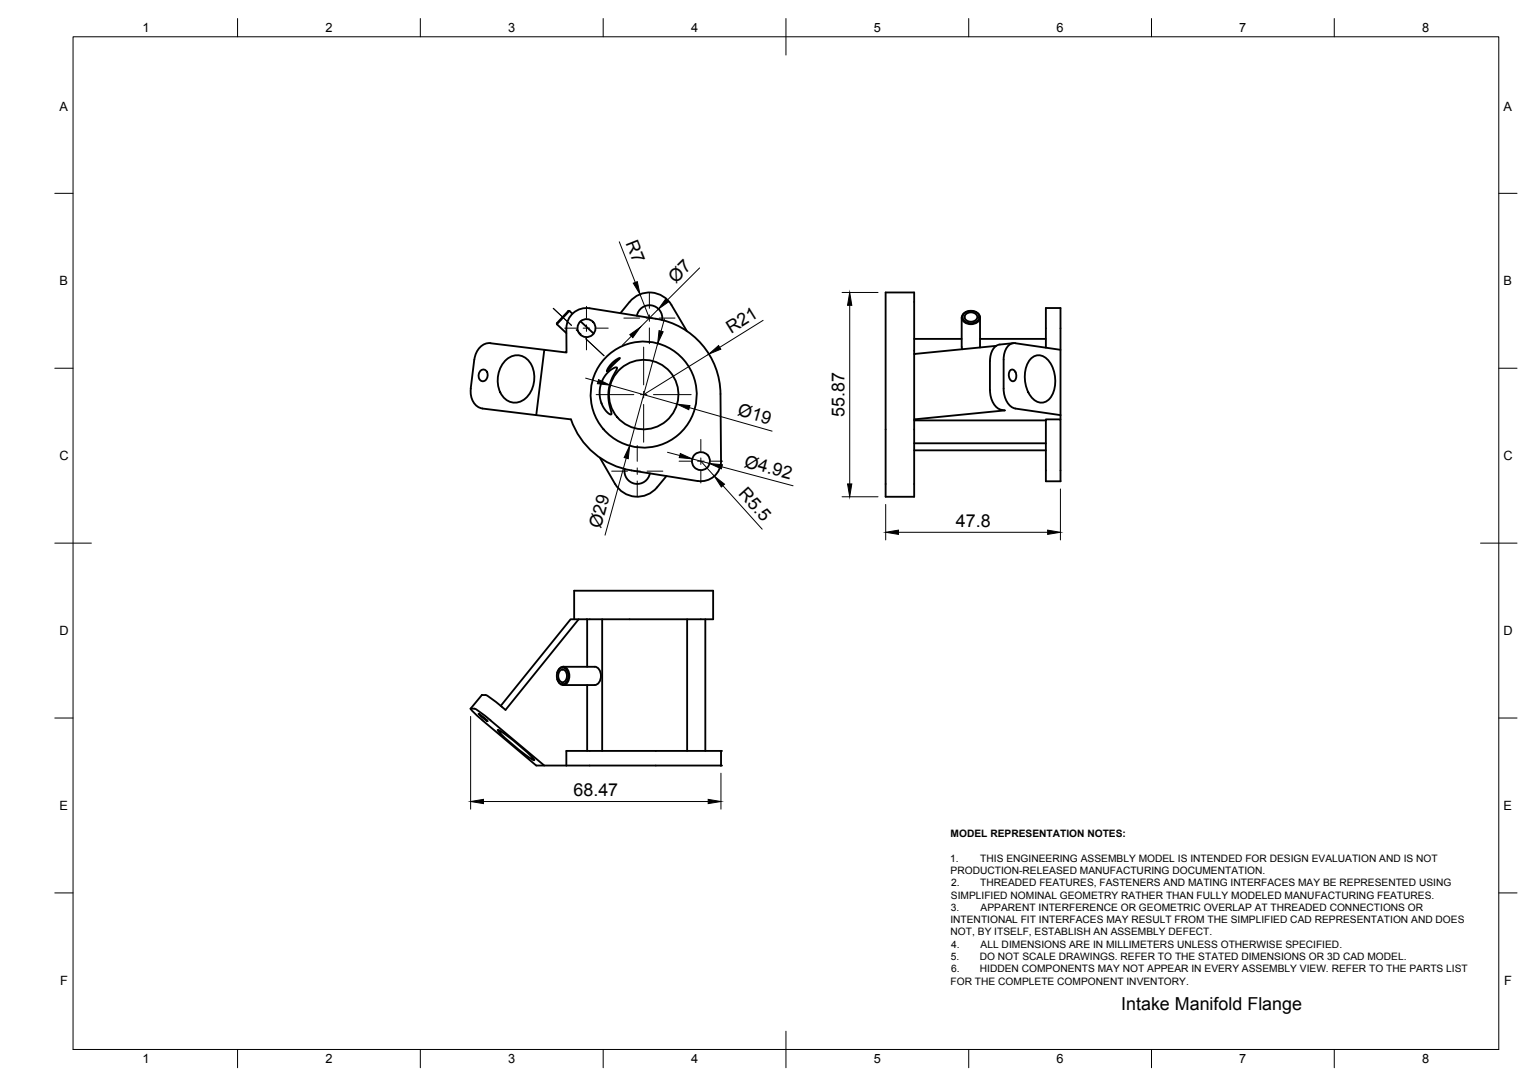
ISO-10303-21;
HEADER;
/* Generated by software containing ST-Developer
 * from STEP Tools, Inc. (www.steptools.com) 
 */

FILE_DESCRIPTION(
/* description */ ('STEP AP214'),
/* implementation_level */ '2;1');

FILE_NAME(
/* name */ 'Intake Manifold Flange.step',
/* time_stamp */ '2026-10-07T12:18:07-07:00',
/* author */ (''),
/* organization */ (''),
/* preprocessor_version */ 'ST-DEVELOPER v20.2',
/* originating_system */ 'Autodesk Translation Framework v15.15.0.0',
/* authorisation */ '');

FILE_SCHEMA (('AUTOMOTIVE_DESIGN { 1 0 10303 214 3 1 1 }'));
ENDSEC;

DATA;
#10=MECHANICAL_DESIGN_GEOMETRIC_PRESENTATION_REPRESENTATION('',(#129),#62974);
#105=SHAPE_REPRESENTATION_RELATIONSHIP('SRR','None',#63028,#117);
#117=ADVANCED_BREP_SHAPE_REPRESENTATION('',(#141),#62969);
#129=STYLED_ITEM('',(#63090),#141);
#141=MANIFOLD_SOLID_BREP('Body1',#15199);
#240=FACE_BOUND('',#5187,.T.);
#241=FACE_BOUND('',#5203,.T.);
#242=FACE_BOUND('',#5205,.T.);
#243=FACE_BOUND('',#5207,.T.);
#244=FACE_BOUND('',#5221,.T.);
#245=FACE_BOUND('',#5223,.T.);
#246=FACE_BOUND('',#5224,.T.);
#247=FACE_BOUND('',#5225,.T.);
#248=FACE_BOUND('',#5228,.T.);
#249=FACE_BOUND('',#5229,.T.);
#250=FACE_BOUND('',#5235,.T.);
#251=FACE_BOUND('',#5236,.T.);
#252=FACE_BOUND('',#5237,.T.);
#253=FACE_BOUND('',#5241,.T.);
#254=FACE_BOUND('',#5242,.T.);
#255=FACE_BOUND('',#5246,.T.);
#256=FACE_BOUND('',#5250,.T.);
#257=FACE_BOUND('',#5253,.T.);
#637=PLANE('',#16431);
#638=PLANE('',#16432);
#639=PLANE('',#16433);
#640=PLANE('',#16434);
#641=PLANE('',#16435);
#642=PLANE('',#16436);
#643=PLANE('',#16437);
#644=PLANE('',#16438);
#645=PLANE('',#16439);
#646=PLANE('',#16443);
#647=PLANE('',#16447);
#648=PLANE('',#16454);
#649=PLANE('',#16455);
#650=PLANE('',#16456);
#651=PLANE('',#16457);
#652=PLANE('',#16458);
#653=PLANE('',#16459);
#654=PLANE('',#16460);
#655=PLANE('',#16462);
#656=PLANE('',#16463);
#657=PLANE('',#16470);
#658=PLANE('',#16471);
#659=PLANE('',#16472);
#660=PLANE('',#16473);
#661=PLANE('',#16474);
#662=PLANE('',#16477);
#663=PLANE('',#16479);
#664=PLANE('',#16480);
#665=PLANE('',#16481);
#666=PLANE('',#16483);
#667=PLANE('',#16484);
#668=PLANE('',#16485);
#912=B_SPLINE_CURVE_WITH_KNOTS('',3,(#45182,#45183,#45184,#45185,#45186,
#45187,#45188,#45189,#45190,#45191,#45192,#45193),.UNSPECIFIED.,.F.,.F.,
(4,2,2,2,2,4),(-1.51152287781019,-1.41955557636733,-1.32295309115156,-1.22686541559156,
-1.13077774003156,-1.03807141782941),.UNSPECIFIED.);
#913=B_SPLINE_CURVE_WITH_KNOTS('',3,(#45198,#45199,#45200,#45201,#45202,
#45203,#45204,#45205,#45206,#45207,#45208,#45209,#45210,#45211,#45212,#45213,
#45214,#45215),.UNSPECIFIED.,.F.,.F.,(4,2,2,2,2,2,2,2,4),(-1.03807141782941,
-1.03415356085079,-0.937529381670028,-0.8405054734841,-0.743481565298172,
-0.650733139326691,-0.55798471335521,-0.464768069683676,-0.459883804363485),
 .UNSPECIFIED.);
#914=B_SPLINE_CURVE_WITH_KNOTS('',3,(#45219,#45220,#45221,#45222,#45223,
#45224,#45225,#45226,#45227,#45228,#45229,#45230,#45231,#45232,#45233),
 .UNSPECIFIED.,.F.,.F.,(4,2,2,2,2,3,4),(-0.459883804363485,-0.371551426012142,
-0.278664247294852,-0.185777068577561,-0.0928885342887805,0.,0.0046338852898157),
 .UNSPECIFIED.);
#915=B_SPLINE_CURVE_WITH_KNOTS('',3,(#45236,#45237,#45238,#45239,#45240,
#45241,#45242,#45243,#45244,#45245,#45246,#45247,#45248,#45249,#45250,#45251,
#45252,#45253,#45254,#45255,#45256,#45257,#45258,#45259,#45260,#45261,#45262,
#45263,#45264,#45265,#45266),.UNSPECIFIED.,.F.,.F.,(4,2,2,3,2,2,2,2,2,2,
2,2,2,2,4),(-1.31063818840695,-1.05024518266218,-0.525122591331091,0.,0.312507098746615,
0.468760648119922,0.62501419749323,0.749593994182574,0.874173790871916,
0.966755699602937,1.05933760833396,1.15191951706498,1.244501425796,1.36908122248534,
1.43505508424711),.UNSPECIFIED.);
#916=B_SPLINE_CURVE_WITH_KNOTS('',3,(#45267,#45268,#45269,#45270,#45271,
#45272,#45273,#45274,#45275,#45276,#45277,#45278,#45279,#45280,#45281,#45282,
#45283,#45284,#45285,#45286,#45287,#45288,#45289,#45290,#45291,#45292),
 .UNSPECIFIED.,.F.,.F.,(4,2,2,2,2,2,2,2,2,2,2,2,4),(1.43505508424711,1.49366101917468,
1.64991456854799,1.8061681179213,2.11867521666791,2.64379780799901,3.1689203993301,
3.67271158289934,3.79227940354027,3.91184722418121,4.03141504482215,4.15098286546309,
4.39438104328756),.UNSPECIFIED.);
#1043=CONICAL_SURFACE('',#16389,14.5,0.104223486416359);
#1044=CONICAL_SURFACE('',#16420,2.5,0.785398163397453);
#1950=LINE('',#45195,#3143);
#1951=LINE('',#45217,#3144);
#1952=LINE('',#45298,#3145);
#1953=LINE('',#45301,#3146);
#1954=LINE('',#45307,#3147);
#1955=LINE('',#45310,#3148);
#1956=LINE('',#45313,#3149);
#1957=LINE('',#45319,#3150);
#1958=LINE('',#45324,#3151);
#1959=LINE('',#45329,#3152);
#1960=LINE('',#45335,#3153);
#1961=LINE('',#45341,#3154);
#1962=LINE('',#45347,#3155);
#1963=LINE('',#45354,#3156);
#1964=LINE('',#45357,#3157);
#1965=LINE('',#45362,#3158);
#1966=LINE('',#45368,#3159);
#1967=LINE('',#45372,#3160);
#1968=LINE('',#45378,#3161);
#1969=LINE('',#45385,#3162);
#1970=LINE('',#45387,#3163);
#1971=LINE('',#45388,#3164);
#1972=LINE('',#45392,#3165);
#1973=LINE('',#45394,#3166);
#1974=LINE('',#45396,#3167);
#1975=LINE('',#45397,#3168);
#1976=LINE('',#45400,#3169);
#1977=LINE('',#45402,#3170);
#1978=LINE('',#45403,#3171);
#1979=LINE('',#45406,#3172);
#1980=LINE('',#45408,#3173);
#1981=LINE('',#45410,#3174);
#1982=LINE('',#45411,#3175);
#1983=LINE('',#45414,#3176);
#1984=LINE('',#45416,#3177);
#1985=LINE('',#45417,#3178);
#1986=LINE('',#45420,#3179);
#1987=LINE('',#45422,#3180);
#1988=LINE('',#45423,#3181);
#1989=LINE('',#45429,#3182);
#1990=LINE('',#45432,#3183);
#1991=LINE('',#45434,#3184);
#1992=LINE('',#45435,#3185);
#1993=LINE('',#45441,#3186);
#1994=LINE('',#45444,#3187);
#1995=LINE('',#45446,#3188);
#1996=LINE('',#45447,#3189);
#1997=LINE('',#45451,#3190);
#1998=LINE('',#45459,#3191);
#1999=LINE('',#45462,#3192);
#2000=LINE('',#45466,#3193);
#2001=LINE('',#45468,#3194);
#2002=LINE('',#45470,#3195);
#2003=LINE('',#45471,#3196);
#2004=LINE('',#45474,#3197);
#2005=LINE('',#45476,#3198);
#2006=LINE('',#45478,#3199);
#2007=LINE('',#45479,#3200);
#2008=LINE('',#45482,#3201);
#2009=LINE('',#45483,#3202);
#2010=LINE('',#45485,#3203);
#2011=LINE('',#45486,#3204);
#2012=LINE('',#45487,#3205);
#2013=LINE('',#45490,#3206);
#2014=LINE('',#45491,#3207);
#2015=LINE('',#45493,#3208);
#2016=LINE('',#45495,#3209);
#2017=LINE('',#45496,#3210);
#2018=LINE('',#45499,#3211);
#2019=LINE('',#45501,#3212);
#2020=LINE('',#45503,#3213);
#2021=LINE('',#45504,#3214);
#2022=LINE('',#45510,#3215);
#2023=LINE('',#45512,#3216);
#2024=LINE('',#45514,#3217);
#2025=LINE('',#45515,#3218);
#2026=LINE('',#45521,#3219);
#2027=LINE('',#45527,#3220);
#2028=LINE('',#45530,#3221);
#2029=LINE('',#45531,#3222);
#2030=LINE('',#45534,#3223);
#2031=LINE('',#45535,#3224);
#2032=LINE('',#45537,#3225);
#2033=LINE('',#45538,#3226);
#2034=LINE('',#45541,#3227);
#2035=LINE('',#45542,#3228);
#2036=LINE('',#45544,#3229);
#2037=LINE('',#45547,#3230);
#2038=LINE('',#45551,#3231);
#2039=LINE('',#45554,#3232);
#2040=LINE('',#45555,#3233);
#2041=LINE('',#45559,#3234);
#2042=LINE('',#45562,#3235);
#2043=LINE('',#45564,#3236);
#3143=VECTOR('',#19955,14.5);
#3144=VECTOR('',#19958,14.5);
#3145=VECTOR('',#19965,1000.);
#3146=VECTOR('',#19968,1000.);
#3147=VECTOR('',#19973,1000.);
#3148=VECTOR('',#19976,1000.);
#3149=VECTOR('',#19979,2.5);
#3150=VECTOR('',#19986,2.4585);
#3151=VECTOR('',#19993,6.5);
#3152=VECTOR('',#19998,1.62099999999999);
#3153=VECTOR('',#20005,2.4585);
#3154=VECTOR('',#20012,3.5);
#3155=VECTOR('',#20019,3.50000000000384);
#3156=VECTOR('',#20026,1000.);
#3157=VECTOR('',#20029,1000.);
#3158=VECTOR('',#20034,2.5);
#3159=VECTOR('',#20041,1.6);
#3160=VECTOR('',#20046,2.5);
#3161=VECTOR('',#20053,1.75);
#3162=VECTOR('',#20064,1000.);
#3163=VECTOR('',#20065,1000.);
#3164=VECTOR('',#20066,1000.);
#3165=VECTOR('',#20069,1000.);
#3166=VECTOR('',#20070,1000.);
#3167=VECTOR('',#20071,1000.);
#3168=VECTOR('',#20072,1000.);
#3169=VECTOR('',#20075,1000.);
#3170=VECTOR('',#20076,1000.);
#3171=VECTOR('',#20077,1000.);
#3172=VECTOR('',#20080,1000.);
#3173=VECTOR('',#20081,1000.);
#3174=VECTOR('',#20082,1000.);
#3175=VECTOR('',#20083,1000.);
#3176=VECTOR('',#20086,1000.);
#3177=VECTOR('',#20087,1000.);
#3178=VECTOR('',#20088,1000.);
#3179=VECTOR('',#20091,1000.);
#3180=VECTOR('',#20092,1000.);
#3181=VECTOR('',#20093,1000.);
#3182=VECTOR('',#20100,1000.);
#3183=VECTOR('',#20103,1000.);
#3184=VECTOR('',#20104,1000.);
#3185=VECTOR('',#20105,1000.);
#3186=VECTOR('',#20112,1000.);
#3187=VECTOR('',#20115,1000.);
#3188=VECTOR('',#20116,1000.);
#3189=VECTOR('',#20117,1000.);
#3190=VECTOR('',#20120,1000.);
#3191=VECTOR('',#20129,1000.);
#3192=VECTOR('',#20132,1000.);
#3193=VECTOR('',#20135,1000.);
#3194=VECTOR('',#20136,1000.);
#3195=VECTOR('',#20137,1000.);
#3196=VECTOR('',#20138,1000.);
#3197=VECTOR('',#20141,1000.);
#3198=VECTOR('',#20142,1000.);
#3199=VECTOR('',#20143,1000.);
#3200=VECTOR('',#20144,1000.);
#3201=VECTOR('',#20147,1000.);
#3202=VECTOR('',#20148,1000.);
#3203=VECTOR('',#20151,1000.);
#3204=VECTOR('',#20152,1000.);
#3205=VECTOR('',#20153,1000.);
#3206=VECTOR('',#20156,1000.);
#3207=VECTOR('',#20157,1000.);
#3208=VECTOR('',#20158,1000.);
#3209=VECTOR('',#20159,1000.);
#3210=VECTOR('',#20160,1000.);
#3211=VECTOR('',#20163,1000.);
#3212=VECTOR('',#20164,1000.);
#3213=VECTOR('',#20165,1000.);
#3214=VECTOR('',#20166,1000.);
#3215=VECTOR('',#20173,1000.);
#3216=VECTOR('',#20174,1000.);
#3217=VECTOR('',#20175,1000.);
#3218=VECTOR('',#20176,1000.);
#3219=VECTOR('',#20183,1000.);
#3220=VECTOR('',#20192,1000.);
#3221=VECTOR('',#20195,1000.);
#3222=VECTOR('',#20196,1000.);
#3223=VECTOR('',#20199,1000.);
#3224=VECTOR('',#20200,1000.);
#3225=VECTOR('',#20201,1000.);
#3226=VECTOR('',#20202,1000.);
#3227=VECTOR('',#20205,1000.);
#3228=VECTOR('',#20206,1000.);
#3229=VECTOR('',#20209,1000.);
#3230=VECTOR('',#20212,1000.);
#3231=VECTOR('',#20219,1000.);
#3232=VECTOR('',#20224,1000.);
#3233=VECTOR('',#20225,1000.);
#3234=VECTOR('',#20230,1000.);
#3235=VECTOR('',#20235,1000.);
#3236=VECTOR('',#20238,1000.);
#3586=CYLINDRICAL_SURFACE('',#16392,5.);
#3587=CYLINDRICAL_SURFACE('',#16395,5.5);
#3588=CYLINDRICAL_SURFACE('',#16398,2.5);
#3589=CYLINDRICAL_SURFACE('',#16400,2.4585);
#3590=CYLINDRICAL_SURFACE('',#16403,6.5);
#3591=CYLINDRICAL_SURFACE('',#16405,1.62099999999999);
#3592=CYLINDRICAL_SURFACE('',#16408,2.4585);
#3593=CYLINDRICAL_SURFACE('',#16411,3.5);
#3594=CYLINDRICAL_SURFACE('',#16414,3.50000000000384);
#3595=CYLINDRICAL_SURFACE('',#16417,7.);
#3596=CYLINDRICAL_SURFACE('',#16423,1.6);
#3597=CYLINDRICAL_SURFACE('',#16426,2.5);
#3598=CYLINDRICAL_SURFACE('',#16428,1.75);
#3599=CYLINDRICAL_SURFACE('',#16440,21.);
#3600=CYLINDRICAL_SURFACE('',#16444,5.5);
#3601=CYLINDRICAL_SURFACE('',#16448,21.);
#3602=CYLINDRICAL_SURFACE('',#16451,5.);
#3603=CYLINDRICAL_SURFACE('',#16467,19.);
#3604=CYLINDRICAL_SURFACE('',#16478,7.00000000000384);
#3605=CYLINDRICAL_SURFACE('',#16487,19.);
#4273=FACE_OUTER_BOUND('',#5186,.T.);
#4274=FACE_OUTER_BOUND('',#5188,.T.);
#4275=FACE_OUTER_BOUND('',#5189,.T.);
#4276=FACE_OUTER_BOUND('',#5190,.T.);
#4277=FACE_OUTER_BOUND('',#5191,.T.);
#4278=FACE_OUTER_BOUND('',#5192,.T.);
#4279=FACE_OUTER_BOUND('',#5193,.T.);
#4280=FACE_OUTER_BOUND('',#5194,.T.);
#4281=FACE_OUTER_BOUND('',#5195,.T.);
#4282=FACE_OUTER_BOUND('',#5196,.T.);
#4283=FACE_OUTER_BOUND('',#5197,.T.);
#4284=FACE_OUTER_BOUND('',#5198,.T.);
#4285=FACE_OUTER_BOUND('',#5199,.T.);
#4286=FACE_OUTER_BOUND('',#5200,.T.);
#4287=FACE_OUTER_BOUND('',#5201,.T.);
#4288=FACE_OUTER_BOUND('',#5202,.T.);
#4289=FACE_OUTER_BOUND('',#5204,.T.);
#4290=FACE_OUTER_BOUND('',#5206,.T.);
#4291=FACE_OUTER_BOUND('',#5208,.T.);
#4292=FACE_OUTER_BOUND('',#5209,.T.);
#4293=FACE_OUTER_BOUND('',#5210,.T.);
#4294=FACE_OUTER_BOUND('',#5211,.T.);
#4295=FACE_OUTER_BOUND('',#5212,.T.);
#4296=FACE_OUTER_BOUND('',#5213,.T.);
#4297=FACE_OUTER_BOUND('',#5214,.T.);
#4298=FACE_OUTER_BOUND('',#5215,.T.);
#4299=FACE_OUTER_BOUND('',#5216,.T.);
#4300=FACE_OUTER_BOUND('',#5217,.T.);
#4301=FACE_OUTER_BOUND('',#5218,.T.);
#4302=FACE_OUTER_BOUND('',#5219,.T.);
#4303=FACE_OUTER_BOUND('',#5220,.T.);
#4304=FACE_OUTER_BOUND('',#5222,.T.);
#4305=FACE_OUTER_BOUND('',#5226,.T.);
#4306=FACE_OUTER_BOUND('',#5227,.T.);
#4307=FACE_OUTER_BOUND('',#5230,.T.);
#4308=FACE_OUTER_BOUND('',#5231,.T.);
#4309=FACE_OUTER_BOUND('',#5232,.T.);
#4310=FACE_OUTER_BOUND('',#5233,.T.);
#4311=FACE_OUTER_BOUND('',#5234,.T.);
#4312=FACE_OUTER_BOUND('',#5238,.T.);
#4313=FACE_OUTER_BOUND('',#5239,.T.);
#4314=FACE_OUTER_BOUND('',#5240,.T.);
#4315=FACE_OUTER_BOUND('',#5243,.T.);
#4316=FACE_OUTER_BOUND('',#5244,.T.);
#4317=FACE_OUTER_BOUND('',#5245,.T.);
#4318=FACE_OUTER_BOUND('',#5247,.T.);
#4319=FACE_OUTER_BOUND('',#5248,.T.);
#4320=FACE_OUTER_BOUND('',#5249,.T.);
#4321=FACE_OUTER_BOUND('',#5251,.T.);
#4322=FACE_OUTER_BOUND('',#5252,.T.);
#4323=FACE_OUTER_BOUND('',#5254,.T.);
#4324=FACE_OUTER_BOUND('',#5255,.T.);
#4325=FACE_OUTER_BOUND('',#5256,.T.);
#4326=FACE_OUTER_BOUND('',#5257,.T.);
#5186=EDGE_LOOP('',(#12825,#12826,#12827,#12828,#12829,#12830,#12831,#12832,
#12833));
#5187=EDGE_LOOP('',(#12834,#12835));
#5188=EDGE_LOOP('',(#12836,#12837,#12838,#12839));
#5189=EDGE_LOOP('',(#12840,#12841,#12842,#12843));
#5190=EDGE_LOOP('',(#12844,#12845,#12846,#12847,#12848,#12849));
#5191=EDGE_LOOP('',(#12850,#12851,#12852,#12853));
#5192=EDGE_LOOP('',(#12854,#12855,#12856,#12857,#12858));
#5193=EDGE_LOOP('',(#12859,#12860,#12861,#12862));
#5194=EDGE_LOOP('',(#12863,#12864,#12865,#12866));
#5195=EDGE_LOOP('',(#12867,#12868,#12869,#12870));
#5196=EDGE_LOOP('',(#12871,#12872,#12873,#12874));
#5197=EDGE_LOOP('',(#12875,#12876,#12877,#12878));
#5198=EDGE_LOOP('',(#12879,#12880,#12881,#12882));
#5199=EDGE_LOOP('',(#12883,#12884,#12885,#12886));
#5200=EDGE_LOOP('',(#12887,#12888,#12889,#12890));
#5201=EDGE_LOOP('',(#12891,#12892,#12893,#12894));
#5202=EDGE_LOOP('',(#12895));
#5203=EDGE_LOOP('',(#12896));
#5204=EDGE_LOOP('',(#12897));
#5205=EDGE_LOOP('',(#12898));
#5206=EDGE_LOOP('',(#12899));
#5207=EDGE_LOOP('',(#12900));
#5208=EDGE_LOOP('',(#12901,#12902,#12903,#12904));
#5209=EDGE_LOOP('',(#12905,#12906,#12907,#12908));
#5210=EDGE_LOOP('',(#12909,#12910,#12911,#12912));
#5211=EDGE_LOOP('',(#12913,#12914,#12915,#12916,#12917));
#5212=EDGE_LOOP('',(#12918,#12919,#12920,#12921));
#5213=EDGE_LOOP('',(#12922,#12923,#12924,#12925));
#5214=EDGE_LOOP('',(#12926,#12927,#12928,#12929));
#5215=EDGE_LOOP('',(#12930,#12931,#12932,#12933));
#5216=EDGE_LOOP('',(#12934,#12935,#12936,#12937));
#5217=EDGE_LOOP('',(#12938,#12939,#12940,#12941));
#5218=EDGE_LOOP('',(#12942,#12943,#12944,#12945));
#5219=EDGE_LOOP('',(#12946,#12947,#12948,#12949));
#5220=EDGE_LOOP('',(#12950,#12951,#12952,#12953));
#5221=EDGE_LOOP('',(#12954));
#5222=EDGE_LOOP('',(#12955,#12956,#12957,#12958,#12959,#12960,#12961,#12962,
#12963,#12964,#12965));
#5223=EDGE_LOOP('',(#12966));
#5224=EDGE_LOOP('',(#12967));
#5225=EDGE_LOOP('',(#12968));
#5226=EDGE_LOOP('',(#12969,#12970,#12971,#12972));
#5227=EDGE_LOOP('',(#12973,#12974,#12975,#12976,#12977,#12978));
#5228=EDGE_LOOP('',(#12979));
#5229=EDGE_LOOP('',(#12980));
#5230=EDGE_LOOP('',(#12981,#12982,#12983,#12984,#12985,#12986,#12987,#12988,
#12989,#12990));
#5231=EDGE_LOOP('',(#12991,#12992,#12993,#12994,#12995));
#5232=EDGE_LOOP('',(#12996,#12997,#12998));
#5233=EDGE_LOOP('',(#12999,#13000,#13001,#13002));
#5234=EDGE_LOOP('',(#13003,#13004,#13005,#13006,#13007,#13008,#13009,#13010));
#5235=EDGE_LOOP('',(#13011));
#5236=EDGE_LOOP('',(#13012));
#5237=EDGE_LOOP('',(#13013));
#5238=EDGE_LOOP('',(#13014,#13015,#13016,#13017,#13018));
#5239=EDGE_LOOP('',(#13019,#13020,#13021,#13022));
#5240=EDGE_LOOP('',(#13023,#13024,#13025,#13026,#13027,#13028,#13029,#13030,
#13031,#13032,#13033,#13034,#13035,#13036,#13037,#13038,#13039));
#5241=EDGE_LOOP('',(#13040));
#5242=EDGE_LOOP('',(#13041));
#5243=EDGE_LOOP('',(#13042,#13043,#13044,#13045));
#5244=EDGE_LOOP('',(#13046,#13047,#13048,#13049,#13050));
#5245=EDGE_LOOP('',(#13051,#13052,#13053,#13054,#13055,#13056,#13057,#13058));
#5246=EDGE_LOOP('',(#13059));
#5247=EDGE_LOOP('',(#13060,#13061,#13062,#13063,#13064));
#5248=EDGE_LOOP('',(#13065,#13066,#13067,#13068));
#5249=EDGE_LOOP('',(#13069,#13070,#13071,#13072,#13073,#13074));
#5250=EDGE_LOOP('',(#13075));
#5251=EDGE_LOOP('',(#13076,#13077,#13078,#13079));
#5252=EDGE_LOOP('',(#13080,#13081,#13082,#13083,#13084,#13085,#13086,#13087,
#13088));
#5253=EDGE_LOOP('',(#13089));
#5254=EDGE_LOOP('',(#13090,#13091,#13092,#13093));
#5255=EDGE_LOOP('',(#13094,#13095,#13096,#13097,#13098,#13099,#13100,#13101,
#13102));
#5256=EDGE_LOOP('',(#13103,#13104,#13105));
#5257=EDGE_LOOP('',(#13106,#13107,#13108,#13109,#13110,#13111,#13112));
#5958=CIRCLE('',#16390,14.5);
#5959=CIRCLE('',#16391,9.5);
#5960=CIRCLE('',#16393,5.);
#5961=CIRCLE('',#16394,5.);
#5962=CIRCLE('',#16396,5.5);
#5963=CIRCLE('',#16397,5.5);
#5964=CIRCLE('',#16399,2.5);
#5965=CIRCLE('',#16401,2.4585);
#5966=CIRCLE('',#16402,2.4585);
#5967=CIRCLE('',#16404,6.5);
#5968=CIRCLE('',#16406,1.621);
#5969=CIRCLE('',#16407,1.621);
#5970=CIRCLE('',#16409,2.4585);
#5971=CIRCLE('',#16410,2.4585);
#5972=CIRCLE('',#16412,3.5);
#5973=CIRCLE('',#16413,3.5);
#5974=CIRCLE('',#16415,3.50000000000384);
#5975=CIRCLE('',#16416,3.50000000000384);
#5976=CIRCLE('',#16418,7.);
#5977=CIRCLE('',#16419,7.);
#5978=CIRCLE('',#16421,2.5);
#5979=CIRCLE('',#16422,2.3);
#5980=CIRCLE('',#16424,1.6);
#5981=CIRCLE('',#16425,1.6);
#5982=CIRCLE('',#16427,2.5);
#5983=CIRCLE('',#16429,1.75);
#5984=CIRCLE('',#16430,1.75);
#5985=CIRCLE('',#16441,21.);
#5986=CIRCLE('',#16442,21.);
#5987=CIRCLE('',#16445,5.5);
#5988=CIRCLE('',#16446,5.5);
#5989=CIRCLE('',#16449,21.);
#5990=CIRCLE('',#16450,21.);
#5991=CIRCLE('',#16452,5.00000000000001);
#5992=CIRCLE('',#16453,5.);
#5993=CIRCLE('',#16461,19.);
#5994=CIRCLE('',#16464,19.);
#5995=CIRCLE('',#16465,7.00000000000384);
#5996=CIRCLE('',#16466,19.);
#5997=CIRCLE('',#16468,19.);
#5998=CIRCLE('',#16469,19.);
#5999=CIRCLE('',#16475,7.00000000000384);
#6000=CIRCLE('',#16476,19.);
#6001=CIRCLE('',#16482,19.);
#6002=CIRCLE('',#16486,19.);
#7176=VERTEX_POINT('',#45180);
#7177=VERTEX_POINT('',#45181);
#7178=VERTEX_POINT('',#45194);
#7179=VERTEX_POINT('',#45197);
#7180=VERTEX_POINT('',#45216);
#7181=VERTEX_POINT('',#45234);
#7182=VERTEX_POINT('',#45235);
#7183=VERTEX_POINT('',#45294);
#7184=VERTEX_POINT('',#45295);
#7185=VERTEX_POINT('',#45297);
#7186=VERTEX_POINT('',#45299);
#7187=VERTEX_POINT('',#45303);
#7188=VERTEX_POINT('',#45304);
#7189=VERTEX_POINT('',#45306);
#7190=VERTEX_POINT('',#45308);
#7191=VERTEX_POINT('',#45312);
#7192=VERTEX_POINT('',#45316);
#7193=VERTEX_POINT('',#45318);
#7194=VERTEX_POINT('',#45322);
#7195=VERTEX_POINT('',#45326);
#7196=VERTEX_POINT('',#45328);
#7197=VERTEX_POINT('',#45332);
#7198=VERTEX_POINT('',#45334);
#7199=VERTEX_POINT('',#45338);
#7200=VERTEX_POINT('',#45340);
#7201=VERTEX_POINT('',#45344);
#7202=VERTEX_POINT('',#45346);
#7203=VERTEX_POINT('',#45350);
#7204=VERTEX_POINT('',#45351);
#7205=VERTEX_POINT('',#45353);
#7206=VERTEX_POINT('',#45355);
#7207=VERTEX_POINT('',#45359);
#7208=VERTEX_POINT('',#45361);
#7209=VERTEX_POINT('',#45365);
#7210=VERTEX_POINT('',#45367);
#7211=VERTEX_POINT('',#45371);
#7212=VERTEX_POINT('',#45375);
#7213=VERTEX_POINT('',#45377);
#7214=VERTEX_POINT('',#45384);
#7215=VERTEX_POINT('',#45386);
#7216=VERTEX_POINT('',#45390);
#7217=VERTEX_POINT('',#45391);
#7218=VERTEX_POINT('',#45393);
#7219=VERTEX_POINT('',#45395);
#7220=VERTEX_POINT('',#45399);
#7221=VERTEX_POINT('',#45401);
#7222=VERTEX_POINT('',#45405);
#7223=VERTEX_POINT('',#45407);
#7224=VERTEX_POINT('',#45409);
#7225=VERTEX_POINT('',#45413);
#7226=VERTEX_POINT('',#45415);
#7227=VERTEX_POINT('',#45419);
#7228=VERTEX_POINT('',#45421);
#7229=VERTEX_POINT('',#45425);
#7230=VERTEX_POINT('',#45427);
#7231=VERTEX_POINT('',#45431);
#7232=VERTEX_POINT('',#45433);
#7233=VERTEX_POINT('',#45437);
#7234=VERTEX_POINT('',#45439);
#7235=VERTEX_POINT('',#45443);
#7236=VERTEX_POINT('',#45445);
#7237=VERTEX_POINT('',#45449);
#7238=VERTEX_POINT('',#45450);
#7239=VERTEX_POINT('',#45455);
#7240=VERTEX_POINT('',#45456);
#7241=VERTEX_POINT('',#45458);
#7242=VERTEX_POINT('',#45460);
#7243=VERTEX_POINT('',#45464);
#7244=VERTEX_POINT('',#45465);
#7245=VERTEX_POINT('',#45467);
#7246=VERTEX_POINT('',#45469);
#7247=VERTEX_POINT('',#45473);
#7248=VERTEX_POINT('',#45475);
#7249=VERTEX_POINT('',#45477);
#7250=VERTEX_POINT('',#45481);
#7251=VERTEX_POINT('',#45489);
#7252=VERTEX_POINT('',#45492);
#7253=VERTEX_POINT('',#45494);
#7254=VERTEX_POINT('',#45498);
#7255=VERTEX_POINT('',#45500);
#7256=VERTEX_POINT('',#45502);
#7257=VERTEX_POINT('',#45508);
#7258=VERTEX_POINT('',#45509);
#7259=VERTEX_POINT('',#45511);
#7260=VERTEX_POINT('',#45513);
#7261=VERTEX_POINT('',#45518);
#7262=VERTEX_POINT('',#45520);
#7263=VERTEX_POINT('',#45524);
#7264=VERTEX_POINT('',#45529);
#7265=VERTEX_POINT('',#45533);
#7266=VERTEX_POINT('',#45536);
#7267=VERTEX_POINT('',#45540);
#7268=VERTEX_POINT('',#45546);
#7269=VERTEX_POINT('',#45558);
#9119=EDGE_CURVE('',#7176,#7177,#912,.F.);
#9120=EDGE_CURVE('',#7176,#7178,#1950,.T.);
#9121=EDGE_CURVE('',#7178,#7178,#5958,.T.);
#9122=EDGE_CURVE('',#7179,#7176,#913,.F.);
#9123=EDGE_CURVE('',#7180,#7179,#1951,.T.);
#9124=EDGE_CURVE('',#7180,#7180,#5959,.T.);
#9125=EDGE_CURVE('',#7177,#7179,#914,.F.);
#9126=EDGE_CURVE('',#7181,#7182,#915,.T.);
#9127=EDGE_CURVE('',#7182,#7181,#916,.T.);
#9128=EDGE_CURVE('',#7183,#7184,#5960,.T.);
#9129=EDGE_CURVE('',#7185,#7183,#1952,.T.);
#9130=EDGE_CURVE('',#7186,#7185,#5961,.T.);
#9131=EDGE_CURVE('',#7184,#7186,#1953,.T.);
#9132=EDGE_CURVE('',#7187,#7188,#5962,.T.);
#9133=EDGE_CURVE('',#7189,#7187,#1954,.T.);
#9134=EDGE_CURVE('',#7189,#7190,#5963,.T.);
#9135=EDGE_CURVE('',#7190,#7188,#1955,.T.);
#9136=EDGE_CURVE('',#7191,#7177,#1956,.T.);
#9137=EDGE_CURVE('',#7191,#7191,#5964,.T.);
#9138=EDGE_CURVE('',#7192,#7192,#5965,.T.);
#9139=EDGE_CURVE('',#7192,#7193,#1957,.T.);
#9140=EDGE_CURVE('',#7193,#7193,#5966,.T.);
#9141=EDGE_CURVE('',#7194,#7194,#5967,.T.);
#9142=EDGE_CURVE('',#7194,#7182,#1958,.T.);
#9143=EDGE_CURVE('',#7195,#7195,#5968,.T.);
#9144=EDGE_CURVE('',#7195,#7196,#1959,.T.);
#9145=EDGE_CURVE('',#7196,#7196,#5969,.T.);
#9146=EDGE_CURVE('',#7197,#7197,#5970,.T.);
#9147=EDGE_CURVE('',#7197,#7198,#1960,.T.);
#9148=EDGE_CURVE('',#7198,#7198,#5971,.T.);
#9149=EDGE_CURVE('',#7199,#7199,#5972,.T.);
#9150=EDGE_CURVE('',#7199,#7200,#1961,.T.);
#9151=EDGE_CURVE('',#7200,#7200,#5973,.T.);
#9152=EDGE_CURVE('',#7201,#7201,#5974,.T.);
#9153=EDGE_CURVE('',#7201,#7202,#1962,.T.);
#9154=EDGE_CURVE('',#7202,#7202,#5975,.T.);
#9155=EDGE_CURVE('',#7203,#7204,#5976,.T.);
#9156=EDGE_CURVE('',#7205,#7204,#1963,.T.);
#9157=EDGE_CURVE('',#7206,#7205,#5977,.T.);
#9158=EDGE_CURVE('',#7206,#7203,#1964,.T.);
#9159=EDGE_CURVE('',#7207,#7207,#5978,.T.);
#9160=EDGE_CURVE('',#7207,#7208,#1965,.T.);
#9161=EDGE_CURVE('',#7208,#7208,#5979,.T.);
#9162=EDGE_CURVE('',#7209,#7209,#5980,.T.);
#9163=EDGE_CURVE('',#7209,#7210,#1966,.T.);
#9164=EDGE_CURVE('',#7210,#7210,#5981,.T.);
#9165=EDGE_CURVE('',#7207,#7211,#1967,.T.);
#9166=EDGE_CURVE('',#7211,#7211,#5982,.T.);
#9167=EDGE_CURVE('',#7212,#7212,#5983,.T.);
#9168=EDGE_CURVE('',#7212,#7213,#1968,.T.);
#9169=EDGE_CURVE('',#7213,#7213,#5984,.T.);
#9170=EDGE_CURVE('',#7214,#7203,#1969,.T.);
#9171=EDGE_CURVE('',#7215,#7206,#1970,.T.);
#9172=EDGE_CURVE('',#7215,#7214,#1971,.T.);
#9173=EDGE_CURVE('',#7216,#7217,#1972,.T.);
#9174=EDGE_CURVE('',#7218,#7216,#1973,.T.);
#9175=EDGE_CURVE('',#7218,#7219,#1974,.T.);
#9176=EDGE_CURVE('',#7219,#7217,#1975,.T.);
#9177=EDGE_CURVE('',#7217,#7220,#1976,.T.);
#9178=EDGE_CURVE('',#7219,#7221,#1977,.T.);
#9179=EDGE_CURVE('',#7221,#7220,#1978,.T.);
#9180=EDGE_CURVE('',#7220,#7222,#1979,.T.);
#9181=EDGE_CURVE('',#7221,#7223,#1980,.T.);
#9182=EDGE_CURVE('',#7223,#7224,#1981,.T.);
#9183=EDGE_CURVE('',#7224,#7222,#1982,.T.);
#9184=EDGE_CURVE('',#7204,#7225,#1983,.T.);
#9185=EDGE_CURVE('',#7226,#7225,#1984,.T.);
#9186=EDGE_CURVE('',#7205,#7226,#1985,.T.);
#9187=EDGE_CURVE('',#7188,#7227,#1986,.T.);
#9188=EDGE_CURVE('',#7190,#7228,#1987,.T.);
#9189=EDGE_CURVE('',#7228,#7227,#1988,.T.);
#9190=EDGE_CURVE('',#7227,#7229,#5985,.T.);
#9191=EDGE_CURVE('',#7228,#7230,#5986,.T.);
#9192=EDGE_CURVE('',#7230,#7229,#1989,.T.);
#9193=EDGE_CURVE('',#7229,#7231,#1990,.T.);
#9194=EDGE_CURVE('',#7230,#7232,#1991,.T.);
#9195=EDGE_CURVE('',#7232,#7231,#1992,.T.);
#9196=EDGE_CURVE('',#7231,#7233,#5987,.T.);
#9197=EDGE_CURVE('',#7232,#7234,#5988,.T.);
#9198=EDGE_CURVE('',#7234,#7233,#1993,.T.);
#9199=EDGE_CURVE('',#7233,#7235,#1994,.T.);
#9200=EDGE_CURVE('',#7234,#7236,#1995,.T.);
#9201=EDGE_CURVE('',#7236,#7235,#1996,.T.);
#9202=EDGE_CURVE('',#7237,#7238,#1997,.T.);
#9203=EDGE_CURVE('',#7235,#7237,#5989,.T.);
#9204=EDGE_CURVE('',#7236,#7238,#5990,.T.);
#9205=EDGE_CURVE('',#7239,#7240,#5991,.T.);
#9206=EDGE_CURVE('',#7241,#7239,#1998,.T.);
#9207=EDGE_CURVE('',#7242,#7241,#5992,.T.);
#9208=EDGE_CURVE('',#7240,#7242,#1999,.T.);
#9209=EDGE_CURVE('',#7243,#7244,#2000,.T.);
#9210=EDGE_CURVE('',#7245,#7243,#2001,.T.);
#9211=EDGE_CURVE('',#7245,#7246,#2002,.T.);
#9212=EDGE_CURVE('',#7246,#7244,#2003,.T.);
#9213=EDGE_CURVE('',#7238,#7247,#2004,.T.);
#9214=EDGE_CURVE('',#7248,#7189,#2005,.T.);
#9215=EDGE_CURVE('',#7248,#7249,#2006,.T.);
#9216=EDGE_CURVE('',#7247,#7249,#2007,.T.);
#9217=EDGE_CURVE('',#7250,#7187,#2008,.T.);
#9218=EDGE_CURVE('',#7250,#7248,#2009,.T.);
#9219=EDGE_CURVE('',#7249,#7186,#2010,.T.);
#9220=EDGE_CURVE('',#7239,#7185,#2011,.T.);
#9221=EDGE_CURVE('',#7247,#7240,#2012,.T.);
#9222=EDGE_CURVE('',#7184,#7251,#2013,.T.);
#9223=EDGE_CURVE('',#7244,#7250,#2014,.T.);
#9224=EDGE_CURVE('',#7252,#7246,#2015,.T.);
#9225=EDGE_CURVE('',#7253,#7252,#2016,.T.);
#9226=EDGE_CURVE('',#7251,#7253,#2017,.T.);
#9227=EDGE_CURVE('',#7254,#7253,#2018,.T.);
#9228=EDGE_CURVE('',#7255,#7254,#2019,.T.);
#9229=EDGE_CURVE('',#7256,#7255,#2020,.T.);
#9230=EDGE_CURVE('',#7256,#7251,#2021,.T.);
#9231=EDGE_CURVE('',#7254,#7252,#5993,.T.);
#9232=EDGE_CURVE('',#7257,#7258,#2022,.T.);
#9233=EDGE_CURVE('',#7259,#7258,#2023,.T.);
#9234=EDGE_CURVE('',#7260,#7259,#2024,.T.);
#9235=EDGE_CURVE('',#7260,#7257,#2025,.T.);
#9236=EDGE_CURVE('',#7226,#7260,#5994,.T.);
#9237=EDGE_CURVE('',#7259,#7261,#5995,.T.);
#9238=EDGE_CURVE('',#7261,#7262,#2026,.T.);
#9239=EDGE_CURVE('',#7262,#7215,#5996,.T.);
#9240=EDGE_CURVE('',#7263,#7223,#5997,.T.);
#9241=EDGE_CURVE('',#7223,#7214,#5998,.T.);
#9242=EDGE_CURVE('',#7262,#7263,#2027,.T.);
#9243=EDGE_CURVE('',#7264,#7263,#2028,.T.);
#9244=EDGE_CURVE('',#7224,#7264,#2029,.T.);
#9245=EDGE_CURVE('',#7265,#7237,#2030,.T.);
#9246=EDGE_CURVE('',#7265,#7216,#2031,.T.);
#9247=EDGE_CURVE('',#7222,#7266,#2032,.T.);
#9248=EDGE_CURVE('',#7266,#7243,#2033,.T.);
#9249=EDGE_CURVE('',#7267,#7266,#2034,.T.);
#9250=EDGE_CURVE('',#7267,#7245,#2035,.T.);
#9251=EDGE_CURVE('',#7264,#7267,#2036,.T.);
#9252=EDGE_CURVE('',#7268,#7264,#2037,.T.);
#9253=EDGE_CURVE('',#7258,#7268,#5999,.T.);
#9254=EDGE_CURVE('',#7252,#7257,#6000,.T.);
#9255=EDGE_CURVE('',#7261,#7268,#2038,.T.);
#9256=EDGE_CURVE('',#7241,#7183,#2039,.T.);
#9257=EDGE_CURVE('',#7242,#7256,#2040,.T.);
#9258=EDGE_CURVE('',#7269,#7218,#2041,.T.);
#9259=EDGE_CURVE('',#7225,#7269,#6001,.T.);
#9260=EDGE_CURVE('',#7269,#7265,#2042,.T.);
#9261=EDGE_CURVE('',#7255,#7269,#2043,.T.);
#9262=EDGE_CURVE('',#7269,#7254,#6002,.T.);
#12825=ORIENTED_EDGE('',*,*,#9119,.F.);
#12826=ORIENTED_EDGE('',*,*,#9120,.T.);
#12827=ORIENTED_EDGE('',*,*,#9121,.F.);
#12828=ORIENTED_EDGE('',*,*,#9120,.F.);
#12829=ORIENTED_EDGE('',*,*,#9122,.F.);
#12830=ORIENTED_EDGE('',*,*,#9123,.F.);
#12831=ORIENTED_EDGE('',*,*,#9124,.T.);
#12832=ORIENTED_EDGE('',*,*,#9123,.T.);
#12833=ORIENTED_EDGE('',*,*,#9125,.F.);
#12834=ORIENTED_EDGE('',*,*,#9126,.F.);
#12835=ORIENTED_EDGE('',*,*,#9127,.F.);
#12836=ORIENTED_EDGE('',*,*,#9128,.F.);
#12837=ORIENTED_EDGE('',*,*,#9129,.F.);
#12838=ORIENTED_EDGE('',*,*,#9130,.F.);
#12839=ORIENTED_EDGE('',*,*,#9131,.F.);
#12840=ORIENTED_EDGE('',*,*,#9132,.F.);
#12841=ORIENTED_EDGE('',*,*,#9133,.F.);
#12842=ORIENTED_EDGE('',*,*,#9134,.T.);
#12843=ORIENTED_EDGE('',*,*,#9135,.T.);
#12844=ORIENTED_EDGE('',*,*,#9136,.F.);
#12845=ORIENTED_EDGE('',*,*,#9137,.F.);
#12846=ORIENTED_EDGE('',*,*,#9136,.T.);
#12847=ORIENTED_EDGE('',*,*,#9125,.T.);
#12848=ORIENTED_EDGE('',*,*,#9122,.T.);
#12849=ORIENTED_EDGE('',*,*,#9119,.T.);
#12850=ORIENTED_EDGE('',*,*,#9138,.T.);
#12851=ORIENTED_EDGE('',*,*,#9139,.T.);
#12852=ORIENTED_EDGE('',*,*,#9140,.T.);
#12853=ORIENTED_EDGE('',*,*,#9139,.F.);
#12854=ORIENTED_EDGE('',*,*,#9141,.F.);
#12855=ORIENTED_EDGE('',*,*,#9142,.T.);
#12856=ORIENTED_EDGE('',*,*,#9127,.T.);
#12857=ORIENTED_EDGE('',*,*,#9126,.T.);
#12858=ORIENTED_EDGE('',*,*,#9142,.F.);
#12859=ORIENTED_EDGE('',*,*,#9143,.T.);
#12860=ORIENTED_EDGE('',*,*,#9144,.T.);
#12861=ORIENTED_EDGE('',*,*,#9145,.F.);
#12862=ORIENTED_EDGE('',*,*,#9144,.F.);
#12863=ORIENTED_EDGE('',*,*,#9146,.T.);
#12864=ORIENTED_EDGE('',*,*,#9147,.T.);
#12865=ORIENTED_EDGE('',*,*,#9148,.T.);
#12866=ORIENTED_EDGE('',*,*,#9147,.F.);
#12867=ORIENTED_EDGE('',*,*,#9149,.T.);
#12868=ORIENTED_EDGE('',*,*,#9150,.T.);
#12869=ORIENTED_EDGE('',*,*,#9151,.F.);
#12870=ORIENTED_EDGE('',*,*,#9150,.F.);
#12871=ORIENTED_EDGE('',*,*,#9152,.T.);
#12872=ORIENTED_EDGE('',*,*,#9153,.T.);
#12873=ORIENTED_EDGE('',*,*,#9154,.F.);
#12874=ORIENTED_EDGE('',*,*,#9153,.F.);
#12875=ORIENTED_EDGE('',*,*,#9155,.T.);
#12876=ORIENTED_EDGE('',*,*,#9156,.F.);
#12877=ORIENTED_EDGE('',*,*,#9157,.F.);
#12878=ORIENTED_EDGE('',*,*,#9158,.T.);
#12879=ORIENTED_EDGE('',*,*,#9159,.F.);
#12880=ORIENTED_EDGE('',*,*,#9160,.T.);
#12881=ORIENTED_EDGE('',*,*,#9161,.F.);
#12882=ORIENTED_EDGE('',*,*,#9160,.F.);
#12883=ORIENTED_EDGE('',*,*,#9162,.F.);
#12884=ORIENTED_EDGE('',*,*,#9163,.T.);
#12885=ORIENTED_EDGE('',*,*,#9164,.T.);
#12886=ORIENTED_EDGE('',*,*,#9163,.F.);
#12887=ORIENTED_EDGE('',*,*,#9159,.T.);
#12888=ORIENTED_EDGE('',*,*,#9165,.T.);
#12889=ORIENTED_EDGE('',*,*,#9166,.F.);
#12890=ORIENTED_EDGE('',*,*,#9165,.F.);
#12891=ORIENTED_EDGE('',*,*,#9167,.F.);
#12892=ORIENTED_EDGE('',*,*,#9168,.T.);
#12893=ORIENTED_EDGE('',*,*,#9169,.T.);
#12894=ORIENTED_EDGE('',*,*,#9168,.F.);
#12895=ORIENTED_EDGE('',*,*,#9161,.T.);
#12896=ORIENTED_EDGE('',*,*,#9167,.T.);
#12897=ORIENTED_EDGE('',*,*,#9169,.F.);
#12898=ORIENTED_EDGE('',*,*,#9164,.F.);
#12899=ORIENTED_EDGE('',*,*,#9137,.T.);
#12900=ORIENTED_EDGE('',*,*,#9162,.T.);
#12901=ORIENTED_EDGE('',*,*,#9170,.T.);
#12902=ORIENTED_EDGE('',*,*,#9158,.F.);
#12903=ORIENTED_EDGE('',*,*,#9171,.F.);
#12904=ORIENTED_EDGE('',*,*,#9172,.T.);
#12905=ORIENTED_EDGE('',*,*,#9173,.F.);
#12906=ORIENTED_EDGE('',*,*,#9174,.F.);
#12907=ORIENTED_EDGE('',*,*,#9175,.T.);
#12908=ORIENTED_EDGE('',*,*,#9176,.T.);
#12909=ORIENTED_EDGE('',*,*,#9177,.F.);
#12910=ORIENTED_EDGE('',*,*,#9176,.F.);
#12911=ORIENTED_EDGE('',*,*,#9178,.T.);
#12912=ORIENTED_EDGE('',*,*,#9179,.T.);
#12913=ORIENTED_EDGE('',*,*,#9180,.F.);
#12914=ORIENTED_EDGE('',*,*,#9179,.F.);
#12915=ORIENTED_EDGE('',*,*,#9181,.T.);
#12916=ORIENTED_EDGE('',*,*,#9182,.T.);
#12917=ORIENTED_EDGE('',*,*,#9183,.T.);
#12918=ORIENTED_EDGE('',*,*,#9184,.T.);
#12919=ORIENTED_EDGE('',*,*,#9185,.F.);
#12920=ORIENTED_EDGE('',*,*,#9186,.F.);
#12921=ORIENTED_EDGE('',*,*,#9156,.T.);
#12922=ORIENTED_EDGE('',*,*,#9187,.F.);
#12923=ORIENTED_EDGE('',*,*,#9135,.F.);
#12924=ORIENTED_EDGE('',*,*,#9188,.T.);
#12925=ORIENTED_EDGE('',*,*,#9189,.T.);
#12926=ORIENTED_EDGE('',*,*,#9190,.F.);
#12927=ORIENTED_EDGE('',*,*,#9189,.F.);
#12928=ORIENTED_EDGE('',*,*,#9191,.T.);
#12929=ORIENTED_EDGE('',*,*,#9192,.T.);
#12930=ORIENTED_EDGE('',*,*,#9193,.F.);
#12931=ORIENTED_EDGE('',*,*,#9192,.F.);
#12932=ORIENTED_EDGE('',*,*,#9194,.T.);
#12933=ORIENTED_EDGE('',*,*,#9195,.T.);
#12934=ORIENTED_EDGE('',*,*,#9196,.F.);
#12935=ORIENTED_EDGE('',*,*,#9195,.F.);
#12936=ORIENTED_EDGE('',*,*,#9197,.T.);
#12937=ORIENTED_EDGE('',*,*,#9198,.T.);
#12938=ORIENTED_EDGE('',*,*,#9199,.F.);
#12939=ORIENTED_EDGE('',*,*,#9198,.F.);
#12940=ORIENTED_EDGE('',*,*,#9200,.T.);
#12941=ORIENTED_EDGE('',*,*,#9201,.T.);
#12942=ORIENTED_EDGE('',*,*,#9202,.F.);
#12943=ORIENTED_EDGE('',*,*,#9203,.F.);
#12944=ORIENTED_EDGE('',*,*,#9201,.F.);
#12945=ORIENTED_EDGE('',*,*,#9204,.T.);
#12946=ORIENTED_EDGE('',*,*,#9205,.F.);
#12947=ORIENTED_EDGE('',*,*,#9206,.F.);
#12948=ORIENTED_EDGE('',*,*,#9207,.F.);
#12949=ORIENTED_EDGE('',*,*,#9208,.F.);
#12950=ORIENTED_EDGE('',*,*,#9209,.F.);
#12951=ORIENTED_EDGE('',*,*,#9210,.F.);
#12952=ORIENTED_EDGE('',*,*,#9211,.T.);
#12953=ORIENTED_EDGE('',*,*,#9212,.T.);
#12954=ORIENTED_EDGE('',*,*,#9166,.T.);
#12955=ORIENTED_EDGE('',*,*,#9213,.F.);
#12956=ORIENTED_EDGE('',*,*,#9204,.F.);
#12957=ORIENTED_EDGE('',*,*,#9200,.F.);
#12958=ORIENTED_EDGE('',*,*,#9197,.F.);
#12959=ORIENTED_EDGE('',*,*,#9194,.F.);
#12960=ORIENTED_EDGE('',*,*,#9191,.F.);
#12961=ORIENTED_EDGE('',*,*,#9188,.F.);
#12962=ORIENTED_EDGE('',*,*,#9134,.F.);
#12963=ORIENTED_EDGE('',*,*,#9214,.F.);
#12964=ORIENTED_EDGE('',*,*,#9215,.T.);
#12965=ORIENTED_EDGE('',*,*,#9216,.F.);
#12966=ORIENTED_EDGE('',*,*,#9121,.T.);
#12967=ORIENTED_EDGE('',*,*,#9138,.F.);
#12968=ORIENTED_EDGE('',*,*,#9146,.F.);
#12969=ORIENTED_EDGE('',*,*,#9217,.F.);
#12970=ORIENTED_EDGE('',*,*,#9218,.T.);
#12971=ORIENTED_EDGE('',*,*,#9214,.T.);
#12972=ORIENTED_EDGE('',*,*,#9133,.T.);
#12973=ORIENTED_EDGE('',*,*,#9219,.T.);
#12974=ORIENTED_EDGE('',*,*,#9130,.T.);
#12975=ORIENTED_EDGE('',*,*,#9220,.F.);
#12976=ORIENTED_EDGE('',*,*,#9205,.T.);
#12977=ORIENTED_EDGE('',*,*,#9221,.F.);
#12978=ORIENTED_EDGE('',*,*,#9216,.T.);
#12979=ORIENTED_EDGE('',*,*,#9141,.T.);
#12980=ORIENTED_EDGE('',*,*,#9143,.F.);
#12981=ORIENTED_EDGE('',*,*,#9222,.F.);
#12982=ORIENTED_EDGE('',*,*,#9131,.T.);
#12983=ORIENTED_EDGE('',*,*,#9219,.F.);
#12984=ORIENTED_EDGE('',*,*,#9215,.F.);
#12985=ORIENTED_EDGE('',*,*,#9218,.F.);
#12986=ORIENTED_EDGE('',*,*,#9223,.F.);
#12987=ORIENTED_EDGE('',*,*,#9212,.F.);
#12988=ORIENTED_EDGE('',*,*,#9224,.F.);
#12989=ORIENTED_EDGE('',*,*,#9225,.F.);
#12990=ORIENTED_EDGE('',*,*,#9226,.F.);
#12991=ORIENTED_EDGE('',*,*,#9226,.T.);
#12992=ORIENTED_EDGE('',*,*,#9227,.F.);
#12993=ORIENTED_EDGE('',*,*,#9228,.F.);
#12994=ORIENTED_EDGE('',*,*,#9229,.F.);
#12995=ORIENTED_EDGE('',*,*,#9230,.T.);
#12996=ORIENTED_EDGE('',*,*,#9225,.T.);
#12997=ORIENTED_EDGE('',*,*,#9231,.F.);
#12998=ORIENTED_EDGE('',*,*,#9227,.T.);
#12999=ORIENTED_EDGE('',*,*,#9232,.T.);
#13000=ORIENTED_EDGE('',*,*,#9233,.F.);
#13001=ORIENTED_EDGE('',*,*,#9234,.F.);
#13002=ORIENTED_EDGE('',*,*,#9235,.T.);
#13003=ORIENTED_EDGE('',*,*,#9186,.T.);
#13004=ORIENTED_EDGE('',*,*,#9236,.T.);
#13005=ORIENTED_EDGE('',*,*,#9234,.T.);
#13006=ORIENTED_EDGE('',*,*,#9237,.T.);
#13007=ORIENTED_EDGE('',*,*,#9238,.T.);
#13008=ORIENTED_EDGE('',*,*,#9239,.T.);
#13009=ORIENTED_EDGE('',*,*,#9171,.T.);
#13010=ORIENTED_EDGE('',*,*,#9157,.T.);
#13011=ORIENTED_EDGE('',*,*,#9152,.F.);
#13012=ORIENTED_EDGE('',*,*,#9149,.F.);
#13013=ORIENTED_EDGE('',*,*,#9124,.F.);
#13014=ORIENTED_EDGE('',*,*,#9240,.T.);
#13015=ORIENTED_EDGE('',*,*,#9241,.T.);
#13016=ORIENTED_EDGE('',*,*,#9172,.F.);
#13017=ORIENTED_EDGE('',*,*,#9239,.F.);
#13018=ORIENTED_EDGE('',*,*,#9242,.T.);
#13019=ORIENTED_EDGE('',*,*,#9240,.F.);
#13020=ORIENTED_EDGE('',*,*,#9243,.F.);
#13021=ORIENTED_EDGE('',*,*,#9244,.F.);
#13022=ORIENTED_EDGE('',*,*,#9182,.F.);
#13023=ORIENTED_EDGE('',*,*,#9245,.F.);
#13024=ORIENTED_EDGE('',*,*,#9246,.T.);
#13025=ORIENTED_EDGE('',*,*,#9173,.T.);
#13026=ORIENTED_EDGE('',*,*,#9177,.T.);
#13027=ORIENTED_EDGE('',*,*,#9180,.T.);
#13028=ORIENTED_EDGE('',*,*,#9247,.T.);
#13029=ORIENTED_EDGE('',*,*,#9248,.T.);
#13030=ORIENTED_EDGE('',*,*,#9209,.T.);
#13031=ORIENTED_EDGE('',*,*,#9223,.T.);
#13032=ORIENTED_EDGE('',*,*,#9217,.T.);
#13033=ORIENTED_EDGE('',*,*,#9132,.T.);
#13034=ORIENTED_EDGE('',*,*,#9187,.T.);
#13035=ORIENTED_EDGE('',*,*,#9190,.T.);
#13036=ORIENTED_EDGE('',*,*,#9193,.T.);
#13037=ORIENTED_EDGE('',*,*,#9196,.T.);
#13038=ORIENTED_EDGE('',*,*,#9199,.T.);
#13039=ORIENTED_EDGE('',*,*,#9203,.T.);
#13040=ORIENTED_EDGE('',*,*,#9140,.F.);
#13041=ORIENTED_EDGE('',*,*,#9148,.F.);
#13042=ORIENTED_EDGE('',*,*,#9248,.F.);
#13043=ORIENTED_EDGE('',*,*,#9249,.F.);
#13044=ORIENTED_EDGE('',*,*,#9250,.T.);
#13045=ORIENTED_EDGE('',*,*,#9210,.T.);
#13046=ORIENTED_EDGE('',*,*,#9247,.F.);
#13047=ORIENTED_EDGE('',*,*,#9183,.F.);
#13048=ORIENTED_EDGE('',*,*,#9244,.T.);
#13049=ORIENTED_EDGE('',*,*,#9251,.T.);
#13050=ORIENTED_EDGE('',*,*,#9249,.T.);
#13051=ORIENTED_EDGE('',*,*,#9224,.T.);
#13052=ORIENTED_EDGE('',*,*,#9211,.F.);
#13053=ORIENTED_EDGE('',*,*,#9250,.F.);
#13054=ORIENTED_EDGE('',*,*,#9251,.F.);
#13055=ORIENTED_EDGE('',*,*,#9252,.F.);
#13056=ORIENTED_EDGE('',*,*,#9253,.F.);
#13057=ORIENTED_EDGE('',*,*,#9232,.F.);
#13058=ORIENTED_EDGE('',*,*,#9254,.F.);
#13059=ORIENTED_EDGE('',*,*,#9154,.T.);
#13060=ORIENTED_EDGE('',*,*,#9252,.T.);
#13061=ORIENTED_EDGE('',*,*,#9243,.T.);
#13062=ORIENTED_EDGE('',*,*,#9242,.F.);
#13063=ORIENTED_EDGE('',*,*,#9238,.F.);
#13064=ORIENTED_EDGE('',*,*,#9255,.T.);
#13065=ORIENTED_EDGE('',*,*,#9253,.T.);
#13066=ORIENTED_EDGE('',*,*,#9255,.F.);
#13067=ORIENTED_EDGE('',*,*,#9237,.F.);
#13068=ORIENTED_EDGE('',*,*,#9233,.T.);
#13069=ORIENTED_EDGE('',*,*,#9256,.T.);
#13070=ORIENTED_EDGE('',*,*,#9128,.T.);
#13071=ORIENTED_EDGE('',*,*,#9222,.T.);
#13072=ORIENTED_EDGE('',*,*,#9230,.F.);
#13073=ORIENTED_EDGE('',*,*,#9257,.F.);
#13074=ORIENTED_EDGE('',*,*,#9207,.T.);
#13075=ORIENTED_EDGE('',*,*,#9145,.T.);
#13076=ORIENTED_EDGE('',*,*,#9220,.T.);
#13077=ORIENTED_EDGE('',*,*,#9129,.T.);
#13078=ORIENTED_EDGE('',*,*,#9256,.F.);
#13079=ORIENTED_EDGE('',*,*,#9206,.T.);
#13080=ORIENTED_EDGE('',*,*,#9181,.F.);
#13081=ORIENTED_EDGE('',*,*,#9178,.F.);
#13082=ORIENTED_EDGE('',*,*,#9175,.F.);
#13083=ORIENTED_EDGE('',*,*,#9258,.F.);
#13084=ORIENTED_EDGE('',*,*,#9259,.F.);
#13085=ORIENTED_EDGE('',*,*,#9184,.F.);
#13086=ORIENTED_EDGE('',*,*,#9155,.F.);
#13087=ORIENTED_EDGE('',*,*,#9170,.F.);
#13088=ORIENTED_EDGE('',*,*,#9241,.F.);
#13089=ORIENTED_EDGE('',*,*,#9151,.T.);
#13090=ORIENTED_EDGE('',*,*,#9246,.F.);
#13091=ORIENTED_EDGE('',*,*,#9260,.F.);
#13092=ORIENTED_EDGE('',*,*,#9258,.T.);
#13093=ORIENTED_EDGE('',*,*,#9174,.T.);
#13094=ORIENTED_EDGE('',*,*,#9221,.T.);
#13095=ORIENTED_EDGE('',*,*,#9208,.T.);
#13096=ORIENTED_EDGE('',*,*,#9257,.T.);
#13097=ORIENTED_EDGE('',*,*,#9229,.T.);
#13098=ORIENTED_EDGE('',*,*,#9261,.T.);
#13099=ORIENTED_EDGE('',*,*,#9260,.T.);
#13100=ORIENTED_EDGE('',*,*,#9245,.T.);
#13101=ORIENTED_EDGE('',*,*,#9202,.T.);
#13102=ORIENTED_EDGE('',*,*,#9213,.T.);
#13103=ORIENTED_EDGE('',*,*,#9228,.T.);
#13104=ORIENTED_EDGE('',*,*,#9262,.F.);
#13105=ORIENTED_EDGE('',*,*,#9261,.F.);
#13106=ORIENTED_EDGE('',*,*,#9259,.T.);
#13107=ORIENTED_EDGE('',*,*,#9262,.T.);
#13108=ORIENTED_EDGE('',*,*,#9231,.T.);
#13109=ORIENTED_EDGE('',*,*,#9254,.T.);
#13110=ORIENTED_EDGE('',*,*,#9235,.F.);
#13111=ORIENTED_EDGE('',*,*,#9236,.F.);
#13112=ORIENTED_EDGE('',*,*,#9185,.T.);
#14908=ADVANCED_FACE('',(#4273,#240),#1043,.F.);
#14909=ADVANCED_FACE('',(#4274),#3586,.T.);
#14910=ADVANCED_FACE('',(#4275),#3587,.T.);
#14911=ADVANCED_FACE('',(#4276),#3588,.F.);
#14912=ADVANCED_FACE('',(#4277),#3589,.F.);
#14913=ADVANCED_FACE('',(#4278),#3590,.F.);
#14914=ADVANCED_FACE('',(#4279),#3591,.F.);
#14915=ADVANCED_FACE('',(#4280),#3592,.F.);
#14916=ADVANCED_FACE('',(#4281),#3593,.F.);
#14917=ADVANCED_FACE('',(#4282),#3594,.F.);
#14918=ADVANCED_FACE('',(#4283),#3595,.T.);
#14919=ADVANCED_FACE('',(#4284),#1044,.T.);
#14920=ADVANCED_FACE('',(#4285),#3596,.F.);
#14921=ADVANCED_FACE('',(#4286),#3597,.T.);
#14922=ADVANCED_FACE('',(#4287),#3598,.F.);
#14923=ADVANCED_FACE('',(#4288,#241),#637,.F.);
#14924=ADVANCED_FACE('',(#4289,#242),#638,.F.);
#14925=ADVANCED_FACE('',(#4290,#243),#639,.T.);
#14926=ADVANCED_FACE('',(#4291),#640,.F.);
#14927=ADVANCED_FACE('',(#4292),#641,.T.);
#14928=ADVANCED_FACE('',(#4293),#642,.T.);
#14929=ADVANCED_FACE('',(#4294),#643,.T.);
#14930=ADVANCED_FACE('',(#4295),#644,.F.);
#14931=ADVANCED_FACE('',(#4296),#645,.T.);
#14932=ADVANCED_FACE('',(#4297),#3599,.T.);
#14933=ADVANCED_FACE('',(#4298),#646,.T.);
#14934=ADVANCED_FACE('',(#4299),#3600,.T.);
#14935=ADVANCED_FACE('',(#4300),#647,.T.);
#14936=ADVANCED_FACE('',(#4301),#3601,.T.);
#14937=ADVANCED_FACE('',(#4302),#3602,.T.);
#14938=ADVANCED_FACE('',(#4303,#244),#648,.T.);
#14939=ADVANCED_FACE('',(#4304,#245,#246,#247),#649,.F.);
#14940=ADVANCED_FACE('',(#4305),#650,.T.);
#14941=ADVANCED_FACE('',(#4306,#248,#249),#651,.F.);
#14942=ADVANCED_FACE('',(#4307),#652,.F.);
#14943=ADVANCED_FACE('',(#4308),#653,.F.);
#14944=ADVANCED_FACE('',(#4309),#654,.F.);
#14945=ADVANCED_FACE('',(#4310),#655,.F.);
#14946=ADVANCED_FACE('',(#4311,#250,#251,#252),#656,.T.);
#14947=ADVANCED_FACE('',(#4312),#3603,.T.);
#14948=ADVANCED_FACE('',(#4313),#657,.F.);
#14949=ADVANCED_FACE('',(#4314,#253,#254),#658,.T.);
#14950=ADVANCED_FACE('',(#4315),#659,.T.);
#14951=ADVANCED_FACE('',(#4316),#660,.T.);
#14952=ADVANCED_FACE('',(#4317,#255),#661,.F.);
#14953=ADVANCED_FACE('',(#4318),#662,.F.);
#14954=ADVANCED_FACE('',(#4319),#3604,.T.);
#14955=ADVANCED_FACE('',(#4320,#256),#663,.F.);
#14956=ADVANCED_FACE('',(#4321),#664,.F.);
#14957=ADVANCED_FACE('',(#4322,#257),#665,.F.);
#14958=ADVANCED_FACE('',(#4323),#666,.T.);
#14959=ADVANCED_FACE('',(#4324),#667,.T.);
#14960=ADVANCED_FACE('',(#4325),#668,.F.);
#14961=ADVANCED_FACE('',(#4326),#3605,.T.);
#15199=CLOSED_SHELL('',(#14908,#14909,#14910,#14911,#14912,#14913,#14914,
#14915,#14916,#14917,#14918,#14919,#14920,#14921,#14922,#14923,#14924,#14925,
#14926,#14927,#14928,#14929,#14930,#14931,#14932,#14933,#14934,#14935,#14936,
#14937,#14938,#14939,#14940,#14941,#14942,#14943,#14944,#14945,#14946,#14947,
#14948,#14949,#14950,#14951,#14952,#14953,#14954,#14955,#14956,#14957,#14958,
#14959,#14960,#14961));
#16388=AXIS2_PLACEMENT_3D('',#45178,#19951,#19952);
#16389=AXIS2_PLACEMENT_3D('',#45179,#19953,#19954);
#16390=AXIS2_PLACEMENT_3D('',#45196,#19956,#19957);
#16391=AXIS2_PLACEMENT_3D('',#45218,#19959,#19960);
#16392=AXIS2_PLACEMENT_3D('',#45293,#19961,#19962);
#16393=AXIS2_PLACEMENT_3D('',#45296,#19963,#19964);
#16394=AXIS2_PLACEMENT_3D('',#45300,#19966,#19967);
#16395=AXIS2_PLACEMENT_3D('',#45302,#19969,#19970);
#16396=AXIS2_PLACEMENT_3D('',#45305,#19971,#19972);
#16397=AXIS2_PLACEMENT_3D('',#45309,#19974,#19975);
#16398=AXIS2_PLACEMENT_3D('',#45311,#19977,#19978);
#16399=AXIS2_PLACEMENT_3D('',#45314,#19980,#19981);
#16400=AXIS2_PLACEMENT_3D('',#45315,#19982,#19983);
#16401=AXIS2_PLACEMENT_3D('',#45317,#19984,#19985);
#16402=AXIS2_PLACEMENT_3D('',#45320,#19987,#19988);
#16403=AXIS2_PLACEMENT_3D('',#45321,#19989,#19990);
#16404=AXIS2_PLACEMENT_3D('',#45323,#19991,#19992);
#16405=AXIS2_PLACEMENT_3D('',#45325,#19994,#19995);
#16406=AXIS2_PLACEMENT_3D('',#45327,#19996,#19997);
#16407=AXIS2_PLACEMENT_3D('',#45330,#19999,#20000);
#16408=AXIS2_PLACEMENT_3D('',#45331,#20001,#20002);
#16409=AXIS2_PLACEMENT_3D('',#45333,#20003,#20004);
#16410=AXIS2_PLACEMENT_3D('',#45336,#20006,#20007);
#16411=AXIS2_PLACEMENT_3D('',#45337,#20008,#20009);
#16412=AXIS2_PLACEMENT_3D('',#45339,#20010,#20011);
#16413=AXIS2_PLACEMENT_3D('',#45342,#20013,#20014);
#16414=AXIS2_PLACEMENT_3D('',#45343,#20015,#20016);
#16415=AXIS2_PLACEMENT_3D('',#45345,#20017,#20018);
#16416=AXIS2_PLACEMENT_3D('',#45348,#20020,#20021);
#16417=AXIS2_PLACEMENT_3D('',#45349,#20022,#20023);
#16418=AXIS2_PLACEMENT_3D('',#45352,#20024,#20025);
#16419=AXIS2_PLACEMENT_3D('',#45356,#20027,#20028);
#16420=AXIS2_PLACEMENT_3D('',#45358,#20030,#20031);
#16421=AXIS2_PLACEMENT_3D('',#45360,#20032,#20033);
#16422=AXIS2_PLACEMENT_3D('',#45363,#20035,#20036);
#16423=AXIS2_PLACEMENT_3D('',#45364,#20037,#20038);
#16424=AXIS2_PLACEMENT_3D('',#45366,#20039,#20040);
#16425=AXIS2_PLACEMENT_3D('',#45369,#20042,#20043);
#16426=AXIS2_PLACEMENT_3D('',#45370,#20044,#20045);
#16427=AXIS2_PLACEMENT_3D('',#45373,#20047,#20048);
#16428=AXIS2_PLACEMENT_3D('',#45374,#20049,#20050);
#16429=AXIS2_PLACEMENT_3D('',#45376,#20051,#20052);
#16430=AXIS2_PLACEMENT_3D('',#45379,#20054,#20055);
#16431=AXIS2_PLACEMENT_3D('',#45380,#20056,#20057);
#16432=AXIS2_PLACEMENT_3D('',#45381,#20058,#20059);
#16433=AXIS2_PLACEMENT_3D('',#45382,#20060,#20061);
#16434=AXIS2_PLACEMENT_3D('',#45383,#20062,#20063);
#16435=AXIS2_PLACEMENT_3D('',#45389,#20067,#20068);
#16436=AXIS2_PLACEMENT_3D('',#45398,#20073,#20074);
#16437=AXIS2_PLACEMENT_3D('',#45404,#20078,#20079);
#16438=AXIS2_PLACEMENT_3D('',#45412,#20084,#20085);
#16439=AXIS2_PLACEMENT_3D('',#45418,#20089,#20090);
#16440=AXIS2_PLACEMENT_3D('',#45424,#20094,#20095);
#16441=AXIS2_PLACEMENT_3D('',#45426,#20096,#20097);
#16442=AXIS2_PLACEMENT_3D('',#45428,#20098,#20099);
#16443=AXIS2_PLACEMENT_3D('',#45430,#20101,#20102);
#16444=AXIS2_PLACEMENT_3D('',#45436,#20106,#20107);
#16445=AXIS2_PLACEMENT_3D('',#45438,#20108,#20109);
#16446=AXIS2_PLACEMENT_3D('',#45440,#20110,#20111);
#16447=AXIS2_PLACEMENT_3D('',#45442,#20113,#20114);
#16448=AXIS2_PLACEMENT_3D('',#45448,#20118,#20119);
#16449=AXIS2_PLACEMENT_3D('',#45452,#20121,#20122);
#16450=AXIS2_PLACEMENT_3D('',#45453,#20123,#20124);
#16451=AXIS2_PLACEMENT_3D('',#45454,#20125,#20126);
#16452=AXIS2_PLACEMENT_3D('',#45457,#20127,#20128);
#16453=AXIS2_PLACEMENT_3D('',#45461,#20130,#20131);
#16454=AXIS2_PLACEMENT_3D('',#45463,#20133,#20134);
#16455=AXIS2_PLACEMENT_3D('',#45472,#20139,#20140);
#16456=AXIS2_PLACEMENT_3D('',#45480,#20145,#20146);
#16457=AXIS2_PLACEMENT_3D('',#45484,#20149,#20150);
#16458=AXIS2_PLACEMENT_3D('',#45488,#20154,#20155);
#16459=AXIS2_PLACEMENT_3D('',#45497,#20161,#20162);
#16460=AXIS2_PLACEMENT_3D('',#45505,#20167,#20168);
#16461=AXIS2_PLACEMENT_3D('',#45506,#20169,#20170);
#16462=AXIS2_PLACEMENT_3D('',#45507,#20171,#20172);
#16463=AXIS2_PLACEMENT_3D('',#45516,#20177,#20178);
#16464=AXIS2_PLACEMENT_3D('',#45517,#20179,#20180);
#16465=AXIS2_PLACEMENT_3D('',#45519,#20181,#20182);
#16466=AXIS2_PLACEMENT_3D('',#45522,#20184,#20185);
#16467=AXIS2_PLACEMENT_3D('',#45523,#20186,#20187);
#16468=AXIS2_PLACEMENT_3D('',#45525,#20188,#20189);
#16469=AXIS2_PLACEMENT_3D('',#45526,#20190,#20191);
#16470=AXIS2_PLACEMENT_3D('',#45528,#20193,#20194);
#16471=AXIS2_PLACEMENT_3D('',#45532,#20197,#20198);
#16472=AXIS2_PLACEMENT_3D('',#45539,#20203,#20204);
#16473=AXIS2_PLACEMENT_3D('',#45543,#20207,#20208);
#16474=AXIS2_PLACEMENT_3D('',#45545,#20210,#20211);
#16475=AXIS2_PLACEMENT_3D('',#45548,#20213,#20214);
#16476=AXIS2_PLACEMENT_3D('',#45549,#20215,#20216);
#16477=AXIS2_PLACEMENT_3D('',#45550,#20217,#20218);
#16478=AXIS2_PLACEMENT_3D('',#45552,#20220,#20221);
#16479=AXIS2_PLACEMENT_3D('',#45553,#20222,#20223);
#16480=AXIS2_PLACEMENT_3D('',#45556,#20226,#20227);
#16481=AXIS2_PLACEMENT_3D('',#45557,#20228,#20229);
#16482=AXIS2_PLACEMENT_3D('',#45560,#20231,#20232);
#16483=AXIS2_PLACEMENT_3D('',#45561,#20233,#20234);
#16484=AXIS2_PLACEMENT_3D('',#45563,#20236,#20237);
#16485=AXIS2_PLACEMENT_3D('',#45565,#20239,#20240);
#16486=AXIS2_PLACEMENT_3D('',#45566,#20241,#20242);
#16487=AXIS2_PLACEMENT_3D('',#45567,#20243,#20244);
#19951=DIRECTION('axis',(0.,0.,1.));
#19952=DIRECTION('refdir',(1.,0.,0.));
#19953=DIRECTION('center_axis',(0.,-1.,0.));
#19954=DIRECTION('ref_axis',(0.,0.,-1.));
#19955=DIRECTION('',(-1.27406007682284E-17,-0.994573647104338,0.104034900324722));
#19956=DIRECTION('center_axis',(0.,1.,0.));
#19957=DIRECTION('ref_axis',(0.645833333333334,0.,-0.763478425075362));
#19958=DIRECTION('',(-1.27406007682284E-17,-0.994573647104339,0.104034900324722));
#19959=DIRECTION('center_axis',(0.,1.,0.));
#19960=DIRECTION('ref_axis',(-0.985799694950984,0.,-0.167925463925357));
#19961=DIRECTION('center_axis',(-0.4309815049242,-0.76811996556279,0.473546894105632));
#19962=DIRECTION('ref_axis',(-5.07348349240606E-16,0.524786664869244,0.85123378479441));
#19963=DIRECTION('center_axis',(0.4309815049242,0.76811996556279,-0.473546894105632));
#19964=DIRECTION('ref_axis',(5.07348349240606E-16,-0.524786664869244,-0.85123378479441));
#19965=DIRECTION('',(0.430981504924199,0.76811996556279,-0.473546894105633));
#19966=DIRECTION('center_axis',(-0.4309815049242,-0.76811996556279,0.473546894105632));
#19967=DIRECTION('ref_axis',(-5.07348349240606E-16,0.524786664869244,0.85123378479441));
#19968=DIRECTION('',(-0.430981504924199,-0.76811996556279,0.473546894105632));
#19969=DIRECTION('center_axis',(0.,-1.,0.));
#19970=DIRECTION('ref_axis',(0.,0.,1.));
#19971=DIRECTION('center_axis',(0.,1.,0.));
#19972=DIRECTION('ref_axis',(1.,0.,0.));
#19973=DIRECTION('',(0.,1.,0.));
#19974=DIRECTION('center_axis',(0.,1.,0.));
#19975=DIRECTION('ref_axis',(1.,0.,0.));
#19976=DIRECTION('',(0.,1.,0.));
#19977=DIRECTION('center_axis',(0.109509747813017,0.,-0.993985721795806));
#19978=DIRECTION('ref_axis',(0.993985721795806,0.,0.109509747813017));
#19979=DIRECTION('',(0.109509747813017,0.,-0.993985721795806));
#19980=DIRECTION('center_axis',(0.109509747813017,0.,-0.993985721795806));
#19981=DIRECTION('ref_axis',(-0.993985721795806,0.,-0.109509747813017));
#19982=DIRECTION('center_axis',(0.,1.,0.));
#19983=DIRECTION('ref_axis',(0.,0.,-1.));
#19984=DIRECTION('center_axis',(0.,-1.,0.));
#19985=DIRECTION('ref_axis',(0.739563468005766,0.,0.673086827081978));
#19986=DIRECTION('',(0.,1.,0.));
#19987=DIRECTION('center_axis',(0.,1.,0.));
#19988=DIRECTION('ref_axis',(0.,0.,1.));
#19989=DIRECTION('center_axis',(0.4309815049242,0.76811996556279,-0.473546894105632));
#19990=DIRECTION('ref_axis',(3.700389135243E-16,-0.524786664869244,-0.85123378479441));
#19991=DIRECTION('center_axis',(0.4309815049242,0.76811996556279,-0.473546894105632));
#19992=DIRECTION('ref_axis',(0.739563468005766,-1.35479487508513E-16,0.673086827081978));
#19993=DIRECTION('',(0.4309815049242,0.76811996556279,-0.473546894105632));
#19994=DIRECTION('center_axis',(0.4309815049242,0.76811996556279,-0.473546894105632));
#19995=DIRECTION('ref_axis',(-2.09125183283633E-15,-0.524786664869243,-0.851233784794411));
#19996=DIRECTION('center_axis',(-0.4309815049242,-0.76811996556279,0.473546894105632));
#19997=DIRECTION('ref_axis',(0.739563468005766,-3.21197772818101E-17,0.673086827081978));
#19998=DIRECTION('',(0.4309815049242,0.76811996556279,-0.473546894105632));
#19999=DIRECTION('center_axis',(-0.4309815049242,-0.76811996556279,0.473546894105632));
#20000=DIRECTION('ref_axis',(7.7903033594954E-16,-0.524786664869244,-0.85123378479441));
#20001=DIRECTION('center_axis',(0.,1.,0.));
#20002=DIRECTION('ref_axis',(0.,0.,-1.));
#20003=DIRECTION('center_axis',(0.,-1.,0.));
#20004=DIRECTION('ref_axis',(0.739563468005766,0.,0.673086827081978));
#20005=DIRECTION('',(0.,1.,0.));
#20006=DIRECTION('center_axis',(0.,1.,0.));
#20007=DIRECTION('ref_axis',(0.,0.,1.));
#20008=DIRECTION('center_axis',(0.,-1.,0.));
#20009=DIRECTION('ref_axis',(0.,0.,1.));
#20010=DIRECTION('center_axis',(0.,1.,0.));
#20011=DIRECTION('ref_axis',(1.,0.,0.));
#20012=DIRECTION('',(0.,-1.,0.));
#20013=DIRECTION('center_axis',(0.,1.,0.));
#20014=DIRECTION('ref_axis',(0.,0.,1.));
#20015=DIRECTION('center_axis',(0.,-1.,0.));
#20016=DIRECTION('ref_axis',(0.,0.,1.));
#20017=DIRECTION('center_axis',(0.,1.,0.));
#20018=DIRECTION('ref_axis',(1.,0.,0.));
#20019=DIRECTION('',(0.,-1.,0.));
#20020=DIRECTION('center_axis',(0.,1.,0.));
#20021=DIRECTION('ref_axis',(0.,0.,1.));
#20022=DIRECTION('center_axis',(0.,1.,0.));
#20023=DIRECTION('ref_axis',(0.,0.,-1.));
#20024=DIRECTION('center_axis',(0.,1.,0.));
#20025=DIRECTION('ref_axis',(1.,0.,0.));
#20026=DIRECTION('',(0.,-1.,0.));
#20027=DIRECTION('center_axis',(0.,1.,0.));
#20028=DIRECTION('ref_axis',(1.,0.,0.));
#20029=DIRECTION('',(0.,-1.,0.));
#20030=DIRECTION('center_axis',(0.109509747813017,0.,-0.993985721795806));
#20031=DIRECTION('ref_axis',(-0.993985721795806,0.,-0.109509747813017));
#20032=DIRECTION('center_axis',(0.109509747813017,0.,-0.993985721795806));
#20033=DIRECTION('ref_axis',(-0.993985721795806,0.,-0.109509747813017));
#20034=DIRECTION('',(-0.780289129569036,8.65956056235497E-17,0.625418958999803));
#20035=DIRECTION('center_axis',(-0.109509747813017,0.,0.993985721795806));
#20036=DIRECTION('ref_axis',(-0.993985721795806,0.,-0.109509747813017));
#20037=DIRECTION('center_axis',(-0.109509747813017,0.,0.993985721795806));
#20038=DIRECTION('ref_axis',(-0.993985721795806,0.,-0.109509747813017));
#20039=DIRECTION('center_axis',(-0.109509747813017,0.,0.993985721795806));
#20040=DIRECTION('ref_axis',(0.993985721795806,0.,0.109509747813017));
#20041=DIRECTION('',(-0.109509747813017,0.,0.993985721795806));
#20042=DIRECTION('center_axis',(-0.109509747813017,0.,0.993985721795806));
#20043=DIRECTION('ref_axis',(0.993985721795806,0.,0.109509747813017));
#20044=DIRECTION('center_axis',(-0.109509747813017,0.,0.993985721795806));
#20045=DIRECTION('ref_axis',(-0.993985721795806,0.,-0.109509747813017));
#20046=DIRECTION('',(0.109509747813017,0.,-0.993985721795806));
#20047=DIRECTION('center_axis',(0.109509747813016,0.,-0.993985721795806));
#20048=DIRECTION('ref_axis',(0.993985721795806,0.,0.109509747813016));
#20049=DIRECTION('center_axis',(0.109509747813017,0.,-0.993985721795806));
#20050=DIRECTION('ref_axis',(0.993985721795806,0.,0.109509747813017));
#20051=DIRECTION('center_axis',(0.109509747813017,0.,-0.993985721795806));
#20052=DIRECTION('ref_axis',(0.993985721795806,0.,0.109509747813017));
#20053=DIRECTION('',(0.109509747813017,0.,-0.993985721795806));
#20054=DIRECTION('center_axis',(0.109509747813017,0.,-0.993985721795806));
#20055=DIRECTION('ref_axis',(0.993985721795806,0.,0.109509747813017));
#20056=DIRECTION('center_axis',(0.109509747813017,0.,-0.993985721795806));
#20057=DIRECTION('ref_axis',(0.,-1.,0.));
#20058=DIRECTION('center_axis',(0.109509747813017,0.,-0.993985721795806));
#20059=DIRECTION('ref_axis',(0.,-1.,0.));
#20060=DIRECTION('center_axis',(0.109509747813017,0.,-0.993985721795806));
#20061=DIRECTION('ref_axis',(0.,-1.,0.));
#20062=DIRECTION('center_axis',(-0.167925463925357,0.,0.985799694950984));
#20063=DIRECTION('ref_axis',(0.,1.,0.));
#20064=DIRECTION('',(-0.985799694950984,0.,-0.167925463925357));
#20065=DIRECTION('',(-0.985799694950984,0.,-0.167925463925357));
#20066=DIRECTION('',(0.,-1.,0.));
#20067=DIRECTION('center_axis',(-0.718304971572534,0.,-0.695728372149779));
#20068=DIRECTION('ref_axis',(-0.695728372149779,0.,0.718304971572534));
#20069=DIRECTION('',(0.695728372149779,0.,-0.718304971572534));
#20070=DIRECTION('',(0.,-1.,0.));
#20071=DIRECTION('',(0.695728372149779,0.,-0.718304971572534));
#20072=DIRECTION('',(0.,-1.,0.));
#20073=DIRECTION('center_axis',(-0.17364817766693,0.,-0.984807753012208));
#20074=DIRECTION('ref_axis',(-0.984807753012208,0.,0.17364817766693));
#20075=DIRECTION('',(0.984807753012208,0.,-0.17364817766693));
#20076=DIRECTION('',(0.984807753012208,0.,-0.17364817766693));
#20077=DIRECTION('',(0.,-1.,0.));
#20078=DIRECTION('center_axis',(0.64278760968654,0.,-0.766044443118978));
#20079=DIRECTION('ref_axis',(0.,-1.,0.));
#20080=DIRECTION('',(0.766044443118978,0.,0.64278760968654));
#20081=DIRECTION('',(0.766044443118978,0.,0.64278760968654));
#20082=DIRECTION('',(0.766044443118978,0.,0.64278760968654));
#20083=DIRECTION('',(0.,-1.,0.));
#20084=DIRECTION('center_axis',(0.982829341293941,0.,-0.184516898661661));
#20085=DIRECTION('ref_axis',(0.,-1.,0.));
#20086=DIRECTION('',(0.184516898661661,0.,0.982829341293941));
#20087=DIRECTION('',(0.,-1.,0.));
#20088=DIRECTION('',(0.184516898661661,0.,0.982829341293941));
#20089=DIRECTION('center_axis',(0.763478425075362,0.,0.645833333333334));
#20090=DIRECTION('ref_axis',(0.,-1.,0.));
#20091=DIRECTION('',(0.645833333333334,0.,-0.763478425075362));
#20092=DIRECTION('',(0.645833333333334,0.,-0.763478425075362));
#20093=DIRECTION('',(0.,1.,0.));
#20094=DIRECTION('center_axis',(0.,-1.,0.));
#20095=DIRECTION('ref_axis',(0.,0.,1.));
#20096=DIRECTION('center_axis',(0.,1.,0.));
#20097=DIRECTION('ref_axis',(-1.,0.,0.));
#20098=DIRECTION('center_axis',(0.,1.,0.));
#20099=DIRECTION('ref_axis',(-1.,0.,0.));
#20100=DIRECTION('',(0.,1.,0.));
#20101=DIRECTION('center_axis',(0.763478425075362,0.,-0.645833333333334));
#20102=DIRECTION('ref_axis',(0.,-1.,0.));
#20103=DIRECTION('',(-0.645833333333334,0.,-0.763478425075362));
#20104=DIRECTION('',(-0.645833333333334,0.,-0.763478425075362));
#20105=DIRECTION('',(0.,1.,0.));
#20106=DIRECTION('center_axis',(0.,-1.,0.));
#20107=DIRECTION('ref_axis',(-1.22464679914735E-16,0.,-1.));
#20108=DIRECTION('center_axis',(0.,1.,0.));
#20109=DIRECTION('ref_axis',(1.,0.,0.));
#20110=DIRECTION('center_axis',(0.,1.,0.));
#20111=DIRECTION('ref_axis',(1.,0.,0.));
#20112=DIRECTION('',(0.,1.,0.));
#20113=DIRECTION('center_axis',(-0.763478425075362,0.,-0.645833333333334));
#20114=DIRECTION('ref_axis',(-0.645833333333334,0.,0.763478425075362));
#20115=DIRECTION('',(-0.645833333333334,0.,0.763478425075362));
#20116=DIRECTION('',(-0.645833333333334,0.,0.763478425075362));
#20117=DIRECTION('',(0.,1.,0.));
#20118=DIRECTION('center_axis',(0.,-1.,0.));
#20119=DIRECTION('ref_axis',(0.,0.,1.));
#20120=DIRECTION('',(0.,-1.,0.));
#20121=DIRECTION('center_axis',(0.,1.,0.));
#20122=DIRECTION('ref_axis',(1.,0.,0.));
#20123=DIRECTION('center_axis',(0.,1.,0.));
#20124=DIRECTION('ref_axis',(1.,0.,0.));
#20125=DIRECTION('center_axis',(0.4309815049242,0.76811996556279,-0.473546894105632));
#20126=DIRECTION('ref_axis',(5.07348349240606E-16,-0.524786664869244,-0.85123378479441));
#20127=DIRECTION('center_axis',(-0.4309815049242,-0.76811996556279,0.473546894105632));
#20128=DIRECTION('ref_axis',(-3.9632604677809E-16,0.524786664869244,0.85123378479441));
#20129=DIRECTION('',(-0.430981504924199,-0.76811996556279,0.473546894105632));
#20130=DIRECTION('center_axis',(0.4309815049242,0.76811996556279,-0.473546894105632));
#20131=DIRECTION('ref_axis',(5.07348349240606E-16,-0.524786664869244,-0.85123378479441));
#20132=DIRECTION('',(0.430981504924199,0.76811996556279,-0.473546894105632));
#20133=DIRECTION('center_axis',(-0.109509747813016,0.,0.993985721795806));
#20134=DIRECTION('ref_axis',(0.,1.,0.));
#20135=DIRECTION('',(-0.993985721795806,0.,-0.109509747813017));
#20136=DIRECTION('',(0.,-1.,0.));
#20137=DIRECTION('',(-0.993985721795806,0.,-0.109509747813017));
#20138=DIRECTION('',(0.,-1.,0.));
#20139=DIRECTION('center_axis',(0.,1.,0.));
#20140=DIRECTION('ref_axis',(1.,0.,0.));
#20141=DIRECTION('',(-0.673086827081978,2.93742993772391E-16,0.739563468005766));
#20142=DIRECTION('',(0.645833333333333,0.,0.763478425075362));
#20143=DIRECTION('',(-0.673086827081978,2.93742993772391E-16,0.739563468005766));
#20144=DIRECTION('',(0.739563468005766,0.,0.673086827081978));
#20145=DIRECTION('center_axis',(-0.763478425075362,0.,0.645833333333334));
#20146=DIRECTION('ref_axis',(0.,1.,0.));
#20147=DIRECTION('',(0.645833333333333,0.,0.763478425075362));
#20148=DIRECTION('',(0.,-1.,0.));
#20149=DIRECTION('center_axis',(0.4309815049242,0.76811996556279,-0.473546894105632));
#20150=DIRECTION('ref_axis',(-0.739563468005766,3.32136590985229E-17,-0.673086827081978));
#20151=DIRECTION('',(-0.517011430438976,0.640305956948566,0.568073465576086));
#20152=DIRECTION('',(0.739563468005766,0.,0.673086827081978));
#20153=DIRECTION('',(-0.517011430438976,0.640305956948566,0.568073465576086));
#20154=DIRECTION('center_axis',(-0.739563468005766,0.,-0.673086827081978));
#20155=DIRECTION('ref_axis',(-0.673086827081978,0.,0.739563468005766));
#20156=DIRECTION('',(0.517011430438976,-0.640305956948566,-0.568073465576087));
#20157=DIRECTION('',(-0.673086827081978,0.,0.739563468005766));
#20158=DIRECTION('',(0.673086827081978,0.,-0.739563468005766));
#20159=DIRECTION('',(0.673086827081978,0.,-0.739563468005766));
#20160=DIRECTION('',(0.424474651014543,0.776076502349984,-0.46639739830567));
#20161=DIRECTION('center_axis',(0.522366870539629,-0.630638773387917,-0.573957829515739));
#20162=DIRECTION('ref_axis',(-1.65075943026669E-17,0.673089942300288,-0.73956063279098));
#20163=DIRECTION('',(0.739563468005766,0.,0.673086827081978));
#20164=DIRECTION('',(0.739563468005766,0.,0.673086827081978));
#20165=DIRECTION('',(0.424474651014543,0.776076502349984,-0.46639739830567));
#20166=DIRECTION('',(0.739563468005766,0.,0.673086827081978));
#20167=DIRECTION('center_axis',(0.,-1.,0.));
#20168=DIRECTION('ref_axis',(0.,0.,-1.));
#20169=DIRECTION('center_axis',(0.,1.,0.));
#20170=DIRECTION('ref_axis',(1.,0.,0.));
#20171=DIRECTION('center_axis',(0.176227439339188,0.,-0.984349475351083));
#20172=DIRECTION('ref_axis',(0.,-1.,0.));
#20173=DIRECTION('',(0.984349475351083,0.,0.176227439339188));
#20174=DIRECTION('',(0.,-1.,0.));
#20175=DIRECTION('',(0.984349475351083,0.,0.176227439339188));
#20176=DIRECTION('',(0.,-1.,0.));
#20177=DIRECTION('center_axis',(0.,1.,0.));
#20178=DIRECTION('ref_axis',(1.,0.,0.));
#20179=DIRECTION('center_axis',(0.,1.,0.));
#20180=DIRECTION('ref_axis',(1.,0.,0.));
#20181=DIRECTION('center_axis',(0.,1.,0.));
#20182=DIRECTION('ref_axis',(-1.,0.,0.));
#20183=DIRECTION('',(-0.176227439496628,0.,-0.984349475322897));
#20184=DIRECTION('center_axis',(0.,1.,0.));
#20185=DIRECTION('ref_axis',(1.,0.,0.));
#20186=DIRECTION('center_axis',(0.,1.,0.));
#20187=DIRECTION('ref_axis',(0.,0.,-1.));
#20188=DIRECTION('center_axis',(0.,1.,0.));
#20189=DIRECTION('ref_axis',(1.,0.,0.));
#20190=DIRECTION('center_axis',(0.,1.,0.));
#20191=DIRECTION('ref_axis',(1.,0.,0.));
#20192=DIRECTION('',(0.,-1.,0.));
#20193=DIRECTION('center_axis',(0.,-1.,0.));
#20194=DIRECTION('ref_axis',(0.,0.,-1.));
#20195=DIRECTION('',(-0.176227439496628,0.,-0.984349475322897));
#20196=DIRECTION('',(0.,0.,1.));
#20197=DIRECTION('center_axis',(0.,1.,0.));
#20198=DIRECTION('ref_axis',(1.,0.,0.));
#20199=DIRECTION('',(-0.673086827081978,0.,0.739563468005766));
#20200=DIRECTION('',(-0.131887341059678,0.,-0.991264712005934));
#20201=DIRECTION('',(0.,0.,1.));
#20202=DIRECTION('',(-0.758169482971429,0.,0.652057539708603));
#20203=DIRECTION('center_axis',(0.652057539708603,0.,0.758169482971429));
#20204=DIRECTION('ref_axis',(0.,-1.,0.));
#20205=DIRECTION('',(0.,-1.,0.));
#20206=DIRECTION('',(-0.758169482971429,0.,0.652057539708603));
#20207=DIRECTION('center_axis',(1.,0.,0.));
#20208=DIRECTION('ref_axis',(0.,1.,0.));
#20209=DIRECTION('',(0.,0.,1.));
#20210=DIRECTION('center_axis',(0.,1.,0.));
#20211=DIRECTION('ref_axis',(1.,0.,0.));
#20212=DIRECTION('',(-0.176227439496628,0.,-0.984349475322897));
#20213=DIRECTION('center_axis',(0.,1.,0.));
#20214=DIRECTION('ref_axis',(-1.,0.,0.));
#20215=DIRECTION('center_axis',(0.,1.,0.));
#20216=DIRECTION('ref_axis',(1.,0.,0.));
#20217=DIRECTION('center_axis',(-0.984349475322897,0.,0.176227439496628));
#20218=DIRECTION('ref_axis',(0.,1.,0.));
#20219=DIRECTION('',(0.,-1.,0.));
#20220=DIRECTION('center_axis',(0.,1.,0.));
#20221=DIRECTION('ref_axis',(0.707106781243096,0.,0.707106781129999));
#20222=DIRECTION('center_axis',(-0.4309815049242,-0.76811996556279,0.473546894105632));
#20223=DIRECTION('ref_axis',(-0.872101888572109,0.489324325932158,-1.43093366045896E-19));
#20224=DIRECTION('',(0.739563468005766,0.,0.673086827081978));
#20225=DIRECTION('',(0.517011430438976,-0.640305956948566,-0.568073465576087));
#20226=DIRECTION('center_axis',(0.517011430438976,-0.640305956948566,-0.568073465576086));
#20227=DIRECTION('ref_axis',(-2.77812299687849E-17,0.663653900301021,-0.748039772081166));
#20228=DIRECTION('center_axis',(0.,1.,0.));
#20229=DIRECTION('ref_axis',(1.,0.,0.));
#20230=DIRECTION('',(-0.131887341059678,0.,-0.991264712005934));
#20231=DIRECTION('center_axis',(0.,1.,0.));
#20232=DIRECTION('ref_axis',(1.,0.,0.));
#20233=DIRECTION('center_axis',(-0.991264712005934,0.,0.131887341059678));
#20234=DIRECTION('ref_axis',(0.,1.,0.));
#20235=DIRECTION('',(0.,-1.,0.));
#20236=DIRECTION('center_axis',(-0.739563468005766,0.,-0.673086827081978));
#20237=DIRECTION('ref_axis',(-0.673086827081978,0.,0.739563468005766));
#20238=DIRECTION('',(0.673086827081978,0.,-0.739563468005766));
#20239=DIRECTION('center_axis',(0.,-1.,0.));
#20240=DIRECTION('ref_axis',(0.,0.,-1.));
#20241=DIRECTION('center_axis',(0.,1.,0.));
#20242=DIRECTION('ref_axis',(1.,0.,0.));
#20243=DIRECTION('center_axis',(0.,1.,0.));
#20244=DIRECTION('ref_axis',(0.,0.,-1.));
#45178=CARTESIAN_POINT('',(0.,0.,0.));
#45179=CARTESIAN_POINT('Origin',(0.,57.,0.));
#45180=CARTESIAN_POINT('',(-1.67399064887303E-12,79.1849791588191,12.1793954854792));
#45181=CARTESIAN_POINT('',(-3.38396588028469,81.4999870102159,11.4475530231091));
#45182=CARTESIAN_POINT('Ctrl Pts',(-3.38396588028469,81.4999870102159,11.4475530231091));
#45183=CARTESIAN_POINT('Ctrl Pts',(-3.38753348202195,81.1933123994846,11.4799495787905));
#45184=CARTESIAN_POINT('Ctrl Pts',(-3.3334689662572,80.8701382063821,11.5316443917672));
#45185=CARTESIAN_POINT('Ctrl Pts',(-3.10178230244334,80.2584031129966,11.6624034476806));
#45186=CARTESIAN_POINT('Ctrl Pts',(-2.91772638565787,79.9722655814763,11.7421072768728));
#45187=CARTESIAN_POINT('Ctrl Pts',(-2.48590576948198,79.5201548688865,11.8893378356882));
#45188=CARTESIAN_POINT('Ctrl Pts',(-2.20964811254668,79.3236980609575,11.9666092782287));
#45189=CARTESIAN_POINT('Ctrl Pts',(-1.59596577782429,79.063039053013,12.0912896144645));
#45190=CARTESIAN_POINT('Ctrl Pts',(-1.25836538845438,78.998920604423,12.1380077071301));
#45191=CARTESIAN_POINT('Ctrl Pts',(-0.63090568596245,79.0010700955652,12.1862255830573));
#45192=CARTESIAN_POINT('Ctrl Pts',(-0.303396633904576,79.0626096753735,
12.1921956406512));
#45193=CARTESIAN_POINT('Ctrl Pts',(-3.35301231224605E-12,79.1849791588191,
12.1793954854792));
#45194=CARTESIAN_POINT('',(-1.77573785876366E-15,57.,14.5));
#45195=CARTESIAN_POINT('',(-1.77573785876366E-15,57.,14.5));
#45196=CARTESIAN_POINT('Origin',(0.,57.,0.));
#45197=CARTESIAN_POINT('',(-2.93399460262726E-12,83.8360320219375,11.6928836797137));
#45198=CARTESIAN_POINT('Ctrl Pts',(-3.35463239703304E-12,79.1849791588191,
12.1793954854792));
#45199=CARTESIAN_POINT('Ctrl Pts',(0.0128218290929213,79.1901506090859,
12.1788545387986));
#45200=CARTESIAN_POINT('Ctrl Pts',(0.0256027230999332,79.1954256888372,
12.1782825024218));
#45201=CARTESIAN_POINT('Ctrl Pts',(0.352471098452155,79.3334249948847,12.1628182515688));
#45202=CARTESIAN_POINT('Ctrl Pts',(0.638723896983974,79.5314817995799,12.1284822027142));
#45203=CARTESIAN_POINT('Ctrl Pts',(1.09095346963654,79.9850955738011,12.0485761528978));
#45204=CARTESIAN_POINT('Ctrl Pts',(1.28733549422776,80.2716995036191,11.997601589275));
#45205=CARTESIAN_POINT('Ctrl Pts',(1.54631117535722,80.8998779199057,11.9007252849027));
#45206=CARTESIAN_POINT('Ctrl Pts',(1.60872112599741,81.241649843226,11.8556144991127));
#45207=CARTESIAN_POINT('Ctrl Pts',(1.59987230256022,81.8707917182341,11.7904023018295));
#45208=CARTESIAN_POINT('Ctrl Pts',(1.53354425429038,82.1986249422797,11.7653209410141));
#45209=CARTESIAN_POINT('Ctrl Pts',(1.27309593871425,82.8002861327028,11.7330462201679));
#45210=CARTESIAN_POINT('Ctrl Pts',(1.0790616457523,83.0741106544731,11.7250993121732));
#45211=CARTESIAN_POINT('Ctrl Pts',(0.634795438436527,83.5062206065111,11.7122867739736));
#45212=CARTESIAN_POINT('Ctrl Pts',(0.354224746857852,83.6933714014299,11.7064436317575));
#45213=CARTESIAN_POINT('Ctrl Pts',(0.0322540850921523,83.8235665140971,
11.6941541060662));
#45214=CARTESIAN_POINT('Ctrl Pts',(0.0161573344640062,83.829883146393,11.6935268675321));
#45215=CARTESIAN_POINT('Ctrl Pts',(-5.86466963477889E-12,83.8360320219375,
11.6928836797137));
#45216=CARTESIAN_POINT('',(-1.16341445918999E-15,104.8,9.5));
#45217=CARTESIAN_POINT('',(-1.77573785876366E-15,57.,14.5));
#45218=CARTESIAN_POINT('Origin',(7.9959910220806E-15,104.8,-1.0842021724855E-15));
#45219=CARTESIAN_POINT('Ctrl Pts',(-5.86329595986257E-12,83.8360320219375,
11.6928836797137));
#45220=CARTESIAN_POINT('Ctrl Pts',(-0.292206849548209,83.9472349901267,
11.6812515700703));
#45221=CARTESIAN_POINT('Ctrl Pts',(-0.605183114261111,84.0009910985821,
11.6636507998233));
#45222=CARTESIAN_POINT('Ctrl Pts',(-1.20746904872849,83.9989278453149,11.6173674315919));
#45223=CARTESIAN_POINT('Ctrl Pts',(-1.53614415691599,83.9368086460649,11.5848936853051));
#45224=CARTESIAN_POINT('Ctrl Pts',(-2.14059633569514,83.6860882677134,11.5152419644677));
#45225=CARTESIAN_POINT('Ctrl Pts',(-2.41645415653066,83.4974908811631,11.4787528322036));
#45226=CARTESIAN_POINT('Ctrl Pts',(-2.85408198422145,83.0627090933434,11.4247140734898));
#45227=CARTESIAN_POINT('Ctrl Pts',(-3.04540036527166,82.7870995589041,11.4036356546425));
#45228=CARTESIAN_POINT('Ctrl Pts',(-3.30525144654228,82.1828149966382,11.3968748343011));
#45229=CARTESIAN_POINT('Ctrl Pts',(-3.37387872914963,81.8541729218928,11.4119012851098));
#45230=CARTESIAN_POINT('Ctrl Pts',(-3.38301135031416,81.5462246274869,11.4427917170341));
#45231=CARTESIAN_POINT('Ctrl Pts',(-3.38346694495989,81.5308621601771,11.4443327330399));
#45232=CARTESIAN_POINT('Ctrl Pts',(-3.38378589319777,81.5154521527978,11.4459193363202));
#45233=CARTESIAN_POINT('Ctrl Pts',(-3.3839657291394,81.4999999999901,11.4475516509024));
#45234=CARTESIAN_POINT('',(-10.2705269140488,83.083888358195,5.75203415488913));
#45235=CARTESIAN_POINT('',(-3.31946532069801,102.294971773814,9.1803280694632));
#45236=CARTESIAN_POINT('Ctrl Pts',(-10.2705269140489,83.0838883581951,5.75203415488913));
#45237=CARTESIAN_POINT('Ctrl Pts',(-10.4476447349629,83.8697062565521,5.26756237969859));
#45238=CARTESIAN_POINT('Ctrl Pts',(-10.5532091788737,84.7143876905477,4.83155183883129));
#45239=CARTESIAN_POINT('Ctrl Pts',(-10.7479632171024,87.0817516344024,3.72991645237086));
#45240=CARTESIAN_POINT('Ctrl Pts',(-10.7473242520368,88.8776077562035,3.06361757662507));
#45241=CARTESIAN_POINT('Ctrl Pts',(-10.594496436306,92.541382067534,2.05817978394714));
#45242=CARTESIAN_POINT('Ctrl Pts',(-10.447233979957,94.4082846127597,1.71460227208681));
#45243=CARTESIAN_POINT('Ctrl Pts',(-10.2675344540495,96.1491949155499,1.68510994751507));
#45244=CARTESIAN_POINT('Ctrl Pts',(-10.1605929923517,97.1852326653713,1.66755869198092));
#45245=CARTESIAN_POINT('Ctrl Pts',(-10.0298236278627,98.3185303401197,1.76805440954025));
#45246=CARTESIAN_POINT('Ctrl Pts',(-9.75871203778378,99.8566120410559,2.26774767596806));
#45247=CARTESIAN_POINT('Ctrl Pts',(-9.65425306299935,100.343635521796,2.49213503112639));
#45248=CARTESIAN_POINT('Ctrl Pts',(-9.39760803176894,101.219568637648,3.04670383868021));
#45249=CARTESIAN_POINT('Ctrl Pts',(-9.2447343379093,101.608464265196,3.37658893604804));
#45250=CARTESIAN_POINT('Ctrl Pts',(-8.9118265271853,102.19936754128,4.02180967320626));
#45251=CARTESIAN_POINT('Ctrl Pts',(-8.72795377133198,102.447311056827,4.35566740291926));
#45252=CARTESIAN_POINT('Ctrl Pts',(-8.30128569109916,102.851557097895,5.04135184709664));
#45253=CARTESIAN_POINT('Ctrl Pts',(-8.057826724156,103.008611139308,5.39232191797367));
#45254=CARTESIAN_POINT('Ctrl Pts',(-7.62991618465407,103.199656130708,5.94403340287079));
#45255=CARTESIAN_POINT('Ctrl Pts',(-7.41696214474173,103.267989331379,6.19847559769947));
#45256=CARTESIAN_POINT('Ctrl Pts',(-6.96343445333318,103.356321073249,6.69063353410446));
#45257=CARTESIAN_POINT('Ctrl Pts',(-6.72278744373644,103.376431260001,6.92826162463383));
#45258=CARTESIAN_POINT('Ctrl Pts',(-6.26631946043173,103.376431260001,7.34369937925353));
#45259=CARTESIAN_POINT('Ctrl Pts',(-6.00714274392577,103.356321073249,7.56096769783146));
#45260=CARTESIAN_POINT('Ctrl Pts',(-5.47456973400649,103.267989331379,7.96627349639138));
#45261=CARTESIAN_POINT('Ctrl Pts',(-5.20125381536694,103.199656130708,8.15439224145004));
#45262=CARTESIAN_POINT('Ctrl Pts',(-4.6117960944632,103.008611139308,8.52860152467425));
#45263=CARTESIAN_POINT('Ctrl Pts',(-4.23951420613461,102.851557097895,8.73802562753481));
#45264=CARTESIAN_POINT('Ctrl Pts',(-3.68678689137256,102.542395564135,9.01364757314303));
#45265=CARTESIAN_POINT('Ctrl Pts',(-3.49844040074224,102.423050920468,9.10136711957112));
#45266=CARTESIAN_POINT('Ctrl Pts',(-3.31946532089988,102.294971773896,9.1803280694126));
#45267=CARTESIAN_POINT('Ctrl Pts',(-3.31946532089987,102.294971773896,9.1803280694126));
#45268=CARTESIAN_POINT('Ctrl Pts',(-3.16047808560999,102.181196440315,9.25047070112544));
#45269=CARTESIAN_POINT('Ctrl Pts',(-3.00889185896816,102.060551508221,9.31375238255998));
#45270=CARTESIAN_POINT('Ctrl Pts',(-2.49351051375685,101.608464265196,9.52097007344027));
#45271=CARTESIAN_POINT('Ctrl Pts',(-2.15072712555426,101.219568637648,9.64218926545221));
#45272=CARTESIAN_POINT('Ctrl Pts',(-1.57450795246704,100.343635521796,9.84562156115182));
#45273=CARTESIAN_POINT('Ctrl Pts',(-1.34130263815093,99.856612041056,9.92854709366551));
#45274=CARTESIAN_POINT('Ctrl Pts',(-0.818357974109837,98.3185303401197,
10.1515352842484));
#45275=CARTESIAN_POINT('Ctrl Pts',(-0.706026039872255,97.1852326653713,
10.2722893835041));
#45276=CARTESIAN_POINT('Ctrl Pts',(-0.725943775135968,94.4082846127598,
10.5620814434823));
#45277=CARTESIAN_POINT('Ctrl Pts',(-1.05417380953003,92.541382067534,10.7409578875094));
#45278=CARTESIAN_POINT('Ctrl Pts',(-2.04081663585263,88.8776077562036,10.9875292351398));
#45279=CARTESIAN_POINT('Ctrl Pts',(-2.70411103697154,87.0817516344024,11.0507363355381));
#45280=CARTESIAN_POINT('Ctrl Pts',(-4.16467604316353,83.9808413773662,10.9322718155721));
#45281=CARTESIAN_POINT('Ctrl Pts',(-5.15529103297173,82.2348877175806,10.7555894278755));
#45282=CARTESIAN_POINT('Ctrl Pts',(-6.55855196256495,80.8708129924728,10.0572521181665));
#45283=CARTESIAN_POINT('Ctrl Pts',(-6.86925488573727,80.6168547487457,9.88291613982572));
#45284=CARTESIAN_POINT('Ctrl Pts',(-7.50690254096133,80.2600262722913,9.45539631479147));
#45285=CARTESIAN_POINT('Ctrl Pts',(-7.83435236046293,80.1604325456248,9.20023978223745));
#45286=CARTESIAN_POINT('Ctrl Pts',(-8.42387230776362,80.1604325456248,8.66370961546201));
#45287=CARTESIAN_POINT('Ctrl Pts',(-8.70865150525079,80.2600262722913,8.36166814633042));
#45288=CARTESIAN_POINT('Ctrl Pts',(-9.19416243184007,80.6168547487457,7.76698598485886));
#45289=CARTESIAN_POINT('Ctrl Pts',(-9.39690556109689,80.8708129924728,7.47402768859298));
#45290=CARTESIAN_POINT('Ctrl Pts',(-9.87846340427557,81.6650788027622,6.69874090289468));
#45291=CARTESIAN_POINT('Ctrl Pts',(-10.1049688770831,82.349357705135,6.20488636169666));
#45292=CARTESIAN_POINT('Ctrl Pts',(-10.2705269140489,83.0838883581951,5.75203415488912));
#45293=CARTESIAN_POINT('Origin',(-26.2797781582403,69.3521366901578,34.6133035514349));
#45294=CARTESIAN_POINT('',(-26.7739714403084,76.2801240271818,35.1563052606437));
#45295=CARTESIAN_POINT('',(-20.4910969480847,73.0785942424389,35.6813720681732));
#45296=CARTESIAN_POINT('Origin',(-24.1889142881135,73.0785942424389,32.3159379327633));
#45297=CARTESIAN_POINT('',(-28.8648353104351,72.5536664749007,37.4536708793154));
#45298=CARTESIAN_POINT('',(-28.8648353104351,72.5536664749007,37.4536708793154));
#45299=CARTESIAN_POINT('',(-22.5819608182114,69.3521366901579,37.9787376868449));
#45300=CARTESIAN_POINT('Origin',(-26.2797781582403,69.3521366901579,34.6133035514349));
#45301=CARTESIAN_POINT('',(-13.4013316692759,85.7143806963486,27.8913943327985));
#45302=CARTESIAN_POINT('Origin',(3.25260651745652E-16,57.,24.));
#45303=CARTESIAN_POINT('',(-4.19913133791449,61.,27.5520833333334));
#45304=CARTESIAN_POINT('',(4.19913133791449,61.,27.5520833333334));
#45305=CARTESIAN_POINT('Origin',(3.25260651745652E-16,61.,24.));
#45306=CARTESIAN_POINT('',(-4.19913133791449,57.,27.5520833333334));
#45307=CARTESIAN_POINT('',(-4.19913133791449,57.,27.5520833333334));
#45308=CARTESIAN_POINT('',(4.19913133791449,57.,27.5520833333334));
#45309=CARTESIAN_POINT('Origin',(3.25260651745652E-16,57.,24.));
#45310=CARTESIAN_POINT('',(4.19913133791449,57.,27.5520833333334));
#45311=CARTESIAN_POINT('Origin',(-0.549839823016682,81.5,8.55209539435995));
#45312=CARTESIAN_POINT('',(-3.48644671444823,81.5,12.3777394943305));
#45313=CARTESIAN_POINT('',(-3.0348041275062,81.5,8.27832102482741));
#45314=CARTESIAN_POINT('Origin',(-1.00148240995872,81.5,12.651513863863));
#45315=CARTESIAN_POINT('Origin',(3.03576608295941E-15,159.117852690362,
24.));
#45316=CARTESIAN_POINT('',(3.33684549852979E-15,57.,26.4585));
#45317=CARTESIAN_POINT('Origin',(3.03576608295941E-15,57.,24.));
#45318=CARTESIAN_POINT('',(3.33684549852979E-15,61.,26.4585));
#45319=CARTESIAN_POINT('',(3.33684549852979E-15,159.117852690362,26.4585));
#45320=CARTESIAN_POINT('Origin',(3.03576608295941E-15,61.,24.));
#45321=CARTESIAN_POINT('Origin',(-0.853633368077759,103.27860563435,0.937941479018354));
#45322=CARTESIAN_POINT('',(-23.6804219928968,66.0065065859266,31.5522110460941));
#45323=CARTESIAN_POINT('Origin',(-23.6804219928968,62.5953932642765,26.0191914449304));
#45324=CARTESIAN_POINT('',(-0.853633368077761,106.689718956,6.47096108018202));
#45325=CARTESIAN_POINT('Origin',(14.1109635503163,148.485307824806,-15.7093526802252));
#45326=CARTESIAN_POINT('',(-29.8584457467901,70.9711830222491,33.98249436695));
#45327=CARTESIAN_POINT('Origin',(-29.8584457467901,70.1205038384961,32.6026444017984));
#45328=CARTESIAN_POINT('',(-27.7675818766634,74.6976405745302,31.6851287482784));
#45329=CARTESIAN_POINT('',(14.1109635503163,149.335987008559,-14.3295027150735));
#45330=CARTESIAN_POINT('Origin',(-27.7675818766633,73.8469613907772,30.3052787831267));
#45331=CARTESIAN_POINT('Origin',(1.3010426069826E-15,159.117852690362,-24.));
#45332=CARTESIAN_POINT('',(1.60212202255298E-15,57.,-21.5415));
#45333=CARTESIAN_POINT('Origin',(1.3010426069826E-15,57.,-24.));
#45334=CARTESIAN_POINT('',(1.60212202255298E-15,61.,-21.5415));
#45335=CARTESIAN_POINT('',(1.60212202255298E-15,159.117852690362,-21.5415));
#45336=CARTESIAN_POINT('Origin',(1.3010426069826E-15,61.,-24.));
#45337=CARTESIAN_POINT('Origin',(-14.9738587466477,89.2,-14.7235713818163));
#45338=CARTESIAN_POINT('',(-14.9738587466477,104.8,-18.2235713818163));
#45339=CARTESIAN_POINT('Origin',(-14.9738587466477,104.8,-14.7235713818163));
#45340=CARTESIAN_POINT('',(-14.9738587466477,97.,-18.2235713818163));
#45341=CARTESIAN_POINT('',(-14.9738587466477,89.2,-18.2235713818163));
#45342=CARTESIAN_POINT('Origin',(-14.9738587466477,97.,-14.7235713818163));
#45343=CARTESIAN_POINT('Origin',(14.8492424010046,89.2,14.8492423986296));
#45344=CARTESIAN_POINT('',(14.8492424010046,104.8,11.3492423986258));
#45345=CARTESIAN_POINT('Origin',(14.8492424010046,104.8,14.8492423986296));
#45346=CARTESIAN_POINT('',(14.8492424010046,97.,11.3492423986258));
#45347=CARTESIAN_POINT('',(14.8492424010046,89.2,11.3492423986258));
#45348=CARTESIAN_POINT('Origin',(14.8492424010046,97.,14.8492423986296));
#45349=CARTESIAN_POINT('Origin',(-14.9738587466477,104.8,-14.7235713818163));
#45350=CARTESIAN_POINT('',(-13.7983804991702,97.,-21.6241692464732));
#45351=CARTESIAN_POINT('',(-21.8536641357053,97.,-13.4319530911847));
#45352=CARTESIAN_POINT('Origin',(-14.9738587466477,97.,-14.7235713818163));
#45353=CARTESIAN_POINT('',(-21.8536641357053,104.8,-13.4319530911847));
#45354=CARTESIAN_POINT('',(-21.8536641357053,104.8,-13.4319530911847));
#45355=CARTESIAN_POINT('',(-13.7983804991702,104.8,-21.6241692464732));
#45356=CARTESIAN_POINT('Origin',(-14.9738587466477,104.8,-14.7235713818163));
#45357=CARTESIAN_POINT('',(-13.7983804991702,104.8,-21.6241692464732));
#45358=CARTESIAN_POINT('Origin',(-2.9507559210307,81.5,30.3444597118283));
#45359=CARTESIAN_POINT('',(-0.465791616541182,81.5,30.6182340813609));
#45360=CARTESIAN_POINT('Origin',(-2.9507559210307,81.5,30.3444597118283));
#45361=CARTESIAN_POINT('',(-0.686490710462955,81.5,30.7951292761574));
#45362=CARTESIAN_POINT('',(-0.465791616541184,81.5,30.6182340813609));
#45363=CARTESIAN_POINT('Origin',(-2.9726578705933,81.5,30.5432568561875));
#45364=CARTESIAN_POINT('Origin',(-1.6585408968371,81.5,18.6154281946378));
#45365=CARTESIAN_POINT('',(0.588894744914294,81.5,12.8267294603638));
#45366=CARTESIAN_POINT('Origin',(-1.001482409959,81.5,12.651513863863));
#45367=CARTESIAN_POINT('',(-0.0681637419638085,81.5,18.7906437911387));
#45368=CARTESIAN_POINT('',(-0.0681637419638084,81.5,18.7906437911387));
#45369=CARTESIAN_POINT('Origin',(-1.6585408968371,81.5,18.6154281946378));
#45370=CARTESIAN_POINT('Origin',(-2.9726578705933,81.5,30.5432568561875));
#45371=CARTESIAN_POINT('',(0.826423407652414,81.5,18.8892025641704));
#45372=CARTESIAN_POINT('',(-0.487693566103787,81.5,30.8170312257201));
#45373=CARTESIAN_POINT('Origin',(-1.6585408968371,81.5,18.6154281946379));
#45374=CARTESIAN_POINT('Origin',(-1.6585408968371,81.5,18.6154281946378));
#45375=CARTESIAN_POINT('',(-4.71213288373597,81.5,30.3516147975147));
#45376=CARTESIAN_POINT('Origin',(-2.9726578705933,81.5,30.5432568561875));
#45377=CARTESIAN_POINT('',(-3.39801590997976,81.5,18.4237861359651));
#45378=CARTESIAN_POINT('',(-3.39801590997976,81.5,18.4237861359651));
#45379=CARTESIAN_POINT('Origin',(-1.6585408968371,81.5,18.6154281946378));
#45380=CARTESIAN_POINT('Origin',(-2.9726578705933,81.5,30.5432568561875));
#45381=CARTESIAN_POINT('Origin',(-1.6585408968371,81.5,18.6154281946378));
#45382=CARTESIAN_POINT('Origin',(-1.001482409959,81.5,12.651513863863));
#45383=CARTESIAN_POINT('Origin',(-13.7983804991702,104.8,-21.6241692464732));
#45384=CARTESIAN_POINT('',(3.19058381458178,97.,-18.7301942040687));
#45385=CARTESIAN_POINT('',(-13.7983804991702,97.,-21.6241692464732));
#45386=CARTESIAN_POINT('',(3.19058381458178,104.8,-18.7301942040687));
#45387=CARTESIAN_POINT('',(-13.7983804991702,104.8,-21.6241692464732));
#45388=CARTESIAN_POINT('',(3.19058381458178,104.8,-18.7301942040687));
#45389=CARTESIAN_POINT('Origin',(-18.9584411954548,97.,-1.25598862991717));
#45390=CARTESIAN_POINT('',(-18.9584411954548,61.,-1.25598862991717));
#45391=CARTESIAN_POINT('',(-4.34139830399414,61.,-16.347359053955));
#45392=CARTESIAN_POINT('',(-18.9584411954548,61.,-1.25598862991717));
#45393=CARTESIAN_POINT('',(-18.9584411954548,97.,-1.25598862991717));
#45394=CARTESIAN_POINT('',(-18.9584411954548,97.,-1.25598862991717));
#45395=CARTESIAN_POINT('',(-4.34139830399414,97.,-16.347359053955));
#45396=CARTESIAN_POINT('',(-18.9584411954548,97.,-1.25598862991717));
#45397=CARTESIAN_POINT('',(-4.34139830399414,97.,-16.347359053955));
#45398=CARTESIAN_POINT('Origin',(2.55225596709131,97.,-17.5628962976236));
#45399=CARTESIAN_POINT('',(2.55225596709131,61.,-17.5628962976236));
#45400=CARTESIAN_POINT('',(2.55225596709131,61.,-17.5628962976236));
#45401=CARTESIAN_POINT('',(2.55225596709131,97.,-17.5628962976236));
#45402=CARTESIAN_POINT('',(2.55225596709131,97.,-17.5628962976236));
#45403=CARTESIAN_POINT('',(2.55225596709131,97.,-17.5628962976236));
#45404=CARTESIAN_POINT('Origin',(18.9542370742857,97.,-3.8));
#45405=CARTESIAN_POINT('',(18.9542370742857,61.,-3.8));
#45406=CARTESIAN_POINT('',(18.9542370742857,61.,-3.8));
#45407=CARTESIAN_POINT('',(18.542188638435,97.,-4.1457496905495));
#45408=CARTESIAN_POINT('',(18.9542370742857,97.,-3.8));
#45409=CARTESIAN_POINT('',(18.9542370742857,97.,-3.8));
#45410=CARTESIAN_POINT('',(18.9542370742857,97.,-3.8));
#45411=CARTESIAN_POINT('',(18.9542370742857,97.,-3.8));
#45412=CARTESIAN_POINT('Origin',(-21.8536641357053,104.8,-13.4319530911847));
#45413=CARTESIAN_POINT('',(-18.6737574845849,97.,3.50582107457153));
#45414=CARTESIAN_POINT('',(-21.8536641357053,97.,-13.4319530911847));
#45415=CARTESIAN_POINT('',(-18.6737574845849,104.8,3.50582107457153));
#45416=CARTESIAN_POINT('',(-18.6737574845849,104.8,3.50582107457153));
#45417=CARTESIAN_POINT('',(-21.8536641357053,104.8,-13.4319530911847));
#45418=CARTESIAN_POINT('Origin',(4.19913133791449,57.,27.5520833333334));
#45419=CARTESIAN_POINT('',(16.0330469265826,61.,13.5625));
#45420=CARTESIAN_POINT('',(4.19913133791449,61.,27.5520833333334));
#45421=CARTESIAN_POINT('',(16.0330469265826,57.,13.5625));
#45422=CARTESIAN_POINT('',(4.19913133791449,57.,27.5520833333334));
#45423=CARTESIAN_POINT('',(16.0330469265826,57.,13.5625));
#45424=CARTESIAN_POINT('Origin',(3.26019593266391E-16,57.,0.));
#45425=CARTESIAN_POINT('',(16.0330469265826,61.,-13.5625));
#45426=CARTESIAN_POINT('Origin',(3.26019593266391E-16,61.,0.));
#45427=CARTESIAN_POINT('',(16.0330469265826,57.,-13.5625));
#45428=CARTESIAN_POINT('Origin',(3.26019593266391E-16,57.,0.));
#45429=CARTESIAN_POINT('',(16.0330469265826,57.,-13.5625));
#45430=CARTESIAN_POINT('Origin',(4.19913133791449,57.,-27.5520833333334));
#45431=CARTESIAN_POINT('',(4.19913133791449,61.,-27.5520833333334));
#45432=CARTESIAN_POINT('',(4.19913133791449,61.,-27.5520833333334));
#45433=CARTESIAN_POINT('',(4.19913133791449,57.,-27.5520833333334));
#45434=CARTESIAN_POINT('',(4.19913133791449,57.,-27.5520833333334));
#45435=CARTESIAN_POINT('',(4.19913133791449,57.,-27.5520833333334));
#45436=CARTESIAN_POINT('Origin',(3.25260651745652E-16,57.,-24.));
#45437=CARTESIAN_POINT('',(-4.19913133791449,61.,-27.5520833333334));
#45438=CARTESIAN_POINT('Origin',(3.25260651745652E-16,61.,-24.));
#45439=CARTESIAN_POINT('',(-4.19913133791449,57.,-27.5520833333334));
#45440=CARTESIAN_POINT('Origin',(3.25260651745652E-16,57.,-24.));
#45441=CARTESIAN_POINT('',(-4.19913133791449,57.,-27.5520833333334));
#45442=CARTESIAN_POINT('Origin',(-16.0330469265826,57.,-13.5625));
#45443=CARTESIAN_POINT('',(-16.0330469265826,61.,-13.5625));
#45444=CARTESIAN_POINT('',(-16.0330469265826,61.,-13.5625));
#45445=CARTESIAN_POINT('',(-16.0330469265826,57.,-13.5625));
#45446=CARTESIAN_POINT('',(-16.0330469265826,57.,-13.5625));
#45447=CARTESIAN_POINT('',(-16.0330469265826,57.,-13.5625));
#45448=CARTESIAN_POINT('Origin',(3.26019593266391E-16,57.,0.));
#45449=CARTESIAN_POINT('',(-19.4844999727208,61.,7.83289606806087));
#45450=CARTESIAN_POINT('',(-19.4844999727208,57.,7.83289606806088));
#45451=CARTESIAN_POINT('',(-19.4844999727208,57.,7.83289606806088));
#45452=CARTESIAN_POINT('Origin',(3.26019593266391E-16,61.,0.));
#45453=CARTESIAN_POINT('Origin',(3.26019593266391E-16,57.,0.));
#45454=CARTESIAN_POINT('Origin',(-23.0156567533509,85.7143806963486,19.1412655807327));
#45455=CARTESIAN_POINT('',(-34.7813430544813,72.5536664749007,32.0689762626596));
#45456=CARTESIAN_POINT('',(-35.8941032423152,69.3521366901579,25.8631747993693));
#45457=CARTESIAN_POINT('Origin',(-32.1962859022864,69.3521366901579,29.2286089347791));
#45458=CARTESIAN_POINT('',(-32.6904791843545,76.2801240271818,29.771610643988));
#45459=CARTESIAN_POINT('',(-34.7813430544813,72.5536664749007,32.0689762626596));
#45460=CARTESIAN_POINT('',(-33.8032393721885,73.0785942424389,23.5658091806977));
#45461=CARTESIAN_POINT('Origin',(-30.1054220321596,73.0785942424389,26.9312433161075));
#45462=CARTESIAN_POINT('',(-33.8032393721885,73.0785942424389,23.5658091806977));
#45463=CARTESIAN_POINT('Origin',(-4.65835823559196,97.,18.2849312538381));
#45464=CARTESIAN_POINT('',(1.34329598298651,61.,18.9461476330332));
#45465=CARTESIAN_POINT('',(-4.65835823559196,61.,18.2849312538381));
#45466=CARTESIAN_POINT('',(-4.65835823559196,61.,18.2849312538381));
#45467=CARTESIAN_POINT('',(1.34329598298651,97.,18.9461476330332));
#45468=CARTESIAN_POINT('',(1.34329598298651,97.,18.9461476330332));
#45469=CARTESIAN_POINT('',(-4.65835823559196,97.,18.2849312538381));
#45470=CARTESIAN_POINT('',(-4.65835823559196,97.,18.2849312538381));
#45471=CARTESIAN_POINT('',(-4.65835823559196,97.,18.2849312538381));
#45472=CARTESIAN_POINT('Origin',(3.25260651745652E-16,57.,24.));
#45473=CARTESIAN_POINT('',(-25.920440199119,57.,14.9044744769683));
#45474=CARTESIAN_POINT('',(-17.9705006596957,57.,6.16936836636249));
#45475=CARTESIAN_POINT('',(-8.48324341658624,57.,22.4875767898433));
#45476=CARTESIAN_POINT('',(-4.19913133791449,57.,27.5520833333334));
#45477=CARTESIAN_POINT('',(-12.6082977750152,57.,27.0200373644439));
#45478=CARTESIAN_POINT('',(-4.65835823559196,57.,18.2849312538381));
#45479=CARTESIAN_POINT('',(-25.920440199119,57.,14.9044744769683));
#45480=CARTESIAN_POINT('Origin',(-4.19913133791449,57.,27.5520833333334));
#45481=CARTESIAN_POINT('',(-8.48324341658624,61.,22.4875767898433));
#45482=CARTESIAN_POINT('',(-4.19913133791449,61.,27.5520833333334));
#45483=CARTESIAN_POINT('',(-8.48324341658624,57.,22.4875767898433));
#45484=CARTESIAN_POINT('Origin',(-25.920440199119,57.,14.9044744769683));
#45485=CARTESIAN_POINT('',(-12.6082977750152,57.,27.0200373644439));
#45486=CARTESIAN_POINT('',(-38.4791603945101,72.5536664749007,28.7035421272497));
#45487=CARTESIAN_POINT('',(-25.920440199119,57.,14.9044744769683));
#45488=CARTESIAN_POINT('Origin',(6.55415551239188,61.,5.96502657159819));
#45489=CARTESIAN_POINT('',(-19.7919116169754,72.2126703843529,34.9131325076166));
#45490=CARTESIAN_POINT('',(-23.0761541002795,76.2801240271818,38.5217393960537));
#45491=CARTESIAN_POINT('',(-5.392814762146,61.,19.0919255286074));
#45492=CARTESIAN_POINT('',(-4.75813954748794,97.,18.3945673514392));
#45493=CARTESIAN_POINT('',(-4.65835823559196,97.,18.2849312538381));
#45494=CARTESIAN_POINT('',(-6.2344942021657,97.,20.0167324637077));
#45495=CARTESIAN_POINT('',(-4.65835823559196,97.,18.2849312538381));
#45496=CARTESIAN_POINT('',(-19.7919116169754,72.2126703843529,34.9131325076166));
#45497=CARTESIAN_POINT('Origin',(-33.1040540410792,72.2126703843529,22.797569620141));
#45498=CARTESIAN_POINT('',(-12.7886497145576,97.,14.0517058921096));
#45499=CARTESIAN_POINT('',(-19.5466366262695,97.,7.90116957623214));
#45500=CARTESIAN_POINT('',(-19.5466366262695,97.,7.90116957623214));
#45501=CARTESIAN_POINT('',(-19.5466366262695,97.,7.90116957623214));
#45502=CARTESIAN_POINT('',(-33.1040540410792,72.2126703843529,22.797569620141));
#45503=CARTESIAN_POINT('',(-33.1040540410792,72.2126703843529,22.797569620141));
#45504=CARTESIAN_POINT('',(-33.1040540410792,72.2126703843529,22.797569620141));
#45505=CARTESIAN_POINT('Origin',(-17.9705006596957,97.,6.16936836636249));
#45506=CARTESIAN_POINT('Origin',(0.,97.,6.93889390390723E-15));
#45507=CARTESIAN_POINT('Origin',(13.6156503256296,104.8,21.7396887260909));
#45508=CARTESIAN_POINT('',(-3.34832134744457,97.,18.7026400316706));
#45509=CARTESIAN_POINT('',(13.6156503256296,97.,21.7396887260909));
#45510=CARTESIAN_POINT('',(13.6156503256296,97.,21.7396887260909));
#45511=CARTESIAN_POINT('',(13.6156503256296,104.8,21.7396887260909));
#45512=CARTESIAN_POINT('',(13.6156503256296,104.8,21.7396887260909));
#45513=CARTESIAN_POINT('',(-3.34832134744457,104.8,18.7026400316706));
#45514=CARTESIAN_POINT('',(13.6156503256296,104.8,21.7396887260909));
#45515=CARTESIAN_POINT('',(-3.34832134744457,104.8,18.7026400316706));
#45516=CARTESIAN_POINT('Origin',(0.,104.8,6.93889390390723E-15));
#45517=CARTESIAN_POINT('Origin',(0.,104.8,6.93889390390723E-15));
#45518=CARTESIAN_POINT('',(21.7396887282687,104.8,13.6156503221525));
#45519=CARTESIAN_POINT('Origin',(14.8492424010046,104.8,14.8492423986296));
#45520=CARTESIAN_POINT('',(18.7026400311351,104.8,-3.34832135043594));
#45521=CARTESIAN_POINT('',(21.7396887282687,104.8,13.6156503221525));
#45522=CARTESIAN_POINT('Origin',(0.,104.8,6.93889390390723E-15));
#45523=CARTESIAN_POINT('Origin',(0.,104.8,6.93889390390723E-15));
#45524=CARTESIAN_POINT('',(18.7026400311351,97.,-3.34832135043594));
#45525=CARTESIAN_POINT('Origin',(0.,97.,6.93889390390723E-15));
#45526=CARTESIAN_POINT('Origin',(0.,97.,6.93889390390723E-15));
#45527=CARTESIAN_POINT('',(18.7026400311351,104.8,-3.34832135043594));
#45528=CARTESIAN_POINT('Origin',(0.,97.,0.));
#45529=CARTESIAN_POINT('',(18.9542370742857,97.,-1.94298164780184));
#45530=CARTESIAN_POINT('',(21.7396887282687,97.,13.6156503221525));
#45531=CARTESIAN_POINT('',(18.9542370742857,97.,3.8));
#45532=CARTESIAN_POINT('Origin',(3.25260651745652E-16,61.,24.));
#45533=CARTESIAN_POINT('',(-17.9705006596957,61.,6.16936836636249));
#45534=CARTESIAN_POINT('',(-18.7049571862498,61.,6.97636264113177));
#45535=CARTESIAN_POINT('',(-17.9705006596957,61.,6.16936836636249));
#45536=CARTESIAN_POINT('',(18.9542370742857,61.,3.8));
#45537=CARTESIAN_POINT('',(18.9542370742857,61.,3.8));
#45538=CARTESIAN_POINT('',(18.9542370742857,61.,3.8));
#45539=CARTESIAN_POINT('Origin',(18.9542370742857,97.,3.8));
#45540=CARTESIAN_POINT('',(18.9542370742857,97.,3.8));
#45541=CARTESIAN_POINT('',(18.9542370742857,97.,3.8));
#45542=CARTESIAN_POINT('',(18.9542370742857,97.,3.8));
#45543=CARTESIAN_POINT('Origin',(18.9542370742857,97.,3.8));
#45544=CARTESIAN_POINT('',(18.9542370742857,97.,3.8));
#45545=CARTESIAN_POINT('Origin',(0.,97.,6.93889390390723E-15));
#45546=CARTESIAN_POINT('',(21.7396887282687,97.,13.6156503221525));
#45547=CARTESIAN_POINT('',(21.7396887282687,97.,13.6156503221525));
#45548=CARTESIAN_POINT('Origin',(14.8492424010046,97.,14.8492423986296));
#45549=CARTESIAN_POINT('Origin',(0.,97.,6.93889390390723E-15));
#45550=CARTESIAN_POINT('Origin',(21.7396887282687,104.8,13.6156503221525));
#45551=CARTESIAN_POINT('',(21.7396887282687,104.8,13.6156503221525));
#45552=CARTESIAN_POINT('Origin',(14.8492424010046,104.8,14.8492423986296));
#45553=CARTESIAN_POINT('Origin',(-36.3882965243833,76.2801240271818,26.4061765085781));
#45554=CARTESIAN_POINT('',(-36.3882965243834,76.2801240271818,26.4061765085781));
#45555=CARTESIAN_POINT('',(-36.3882965243833,76.2801240271818,26.4061765085781));
#45556=CARTESIAN_POINT('Origin',(-38.4791603945101,72.5536664749007,28.7035421272497));
#45557=CARTESIAN_POINT('Origin',(0.,97.,6.93889390390723E-15));
#45558=CARTESIAN_POINT('',(-17.9705006596957,97.,6.16936836636249));
#45559=CARTESIAN_POINT('',(-17.9705006596957,97.,6.16936836636249));
#45560=CARTESIAN_POINT('Origin',(0.,97.,6.93889390390723E-15));
#45561=CARTESIAN_POINT('Origin',(-17.9705006596957,97.,6.16936836636249));
#45562=CARTESIAN_POINT('',(-17.9705006596957,97.,6.16936836636249));
#45563=CARTESIAN_POINT('Origin',(-6.75798691171192,61.,-6.15053631587742));
#45564=CARTESIAN_POINT('',(-17.9705006596957,97.,6.16936836636249));
#45565=CARTESIAN_POINT('Origin',(-17.9705006596957,97.,6.16936836636249));
#45566=CARTESIAN_POINT('Origin',(0.,97.,6.93889390390723E-15));
#45567=CARTESIAN_POINT('Origin',(0.,104.8,6.93889390390723E-15));
#62955=UNCERTAINTY_MEASURE_WITH_UNIT(LENGTH_MEASURE(0.01),#62975,
'DISTANCE_ACCURACY_VALUE',
'Maximum model space distance between geometric entities at asserted c
onnectivities');
#62960=UNCERTAINTY_MEASURE_WITH_UNIT(LENGTH_MEASURE(0.01),#62975,
'DISTANCE_ACCURACY_VALUE',
'Maximum model space distance between geometric entities at asserted c
onnectivities');
#62969=(
GEOMETRIC_REPRESENTATION_CONTEXT(3)
GLOBAL_UNCERTAINTY_ASSIGNED_CONTEXT((#62955))
GLOBAL_UNIT_ASSIGNED_CONTEXT((#62975,#62977,#62978))
REPRESENTATION_CONTEXT('','3D')
);
#62974=(
GEOMETRIC_REPRESENTATION_CONTEXT(3)
GLOBAL_UNCERTAINTY_ASSIGNED_CONTEXT((#62960))
GLOBAL_UNIT_ASSIGNED_CONTEXT((#62975,#62977,#62978))
REPRESENTATION_CONTEXT('','3D')
);
#62975=(
LENGTH_UNIT()
NAMED_UNIT(*)
SI_UNIT(.MILLI.,.METRE.)
);
#62977=(
NAMED_UNIT(*)
PLANE_ANGLE_UNIT()
SI_UNIT($,.RADIAN.)
);
#62978=(
NAMED_UNIT(*)
SI_UNIT($,.STERADIAN.)
SOLID_ANGLE_UNIT()
);
#62987=SHAPE_DEFINITION_REPRESENTATION(#63000,#63028);
#63000=PRODUCT_DEFINITION_SHAPE('',$,#63042);
#63028=SHAPE_REPRESENTATION('',(#16388),#62969);
#63033=PRODUCT_DEFINITION_CONTEXT('part definition',#63074,'design');
#63042=PRODUCT_DEFINITION('Intake Manifold Flange',
'Intake Manifold Flange',#63055,#63033);
#63055=PRODUCT_DEFINITION_FORMATION('',$,#63084);
#63074=APPLICATION_CONTEXT(
'Core Data for Automotive Mechanical Design Process');
#63075=PRODUCT_CONTEXT('part definition',#63074,'mechanical');
#63084=PRODUCT('Intake Manifold Flange','Intake Manifold Flange',$,(#63075));
#63090=PRESENTATION_STYLE_ASSIGNMENT((#63092));
#63092=SURFACE_STYLE_USAGE(.BOTH.,#63094);
#63094=SURFACE_SIDE_STYLE('',(#63096));
#63096=SURFACE_STYLE_FILL_AREA(#63098);
#63098=FILL_AREA_STYLE('Opaque(202,209,238)',(#63100));
#63100=FILL_AREA_STYLE_COLOUR('Opaque(202,209,238)',#63102);
#63102=COLOUR_RGB('Opaque(202,209,238)', 0.66274510, 0.83137255, 0.94901961);
ENDSEC;
END-ISO-10303-21;
